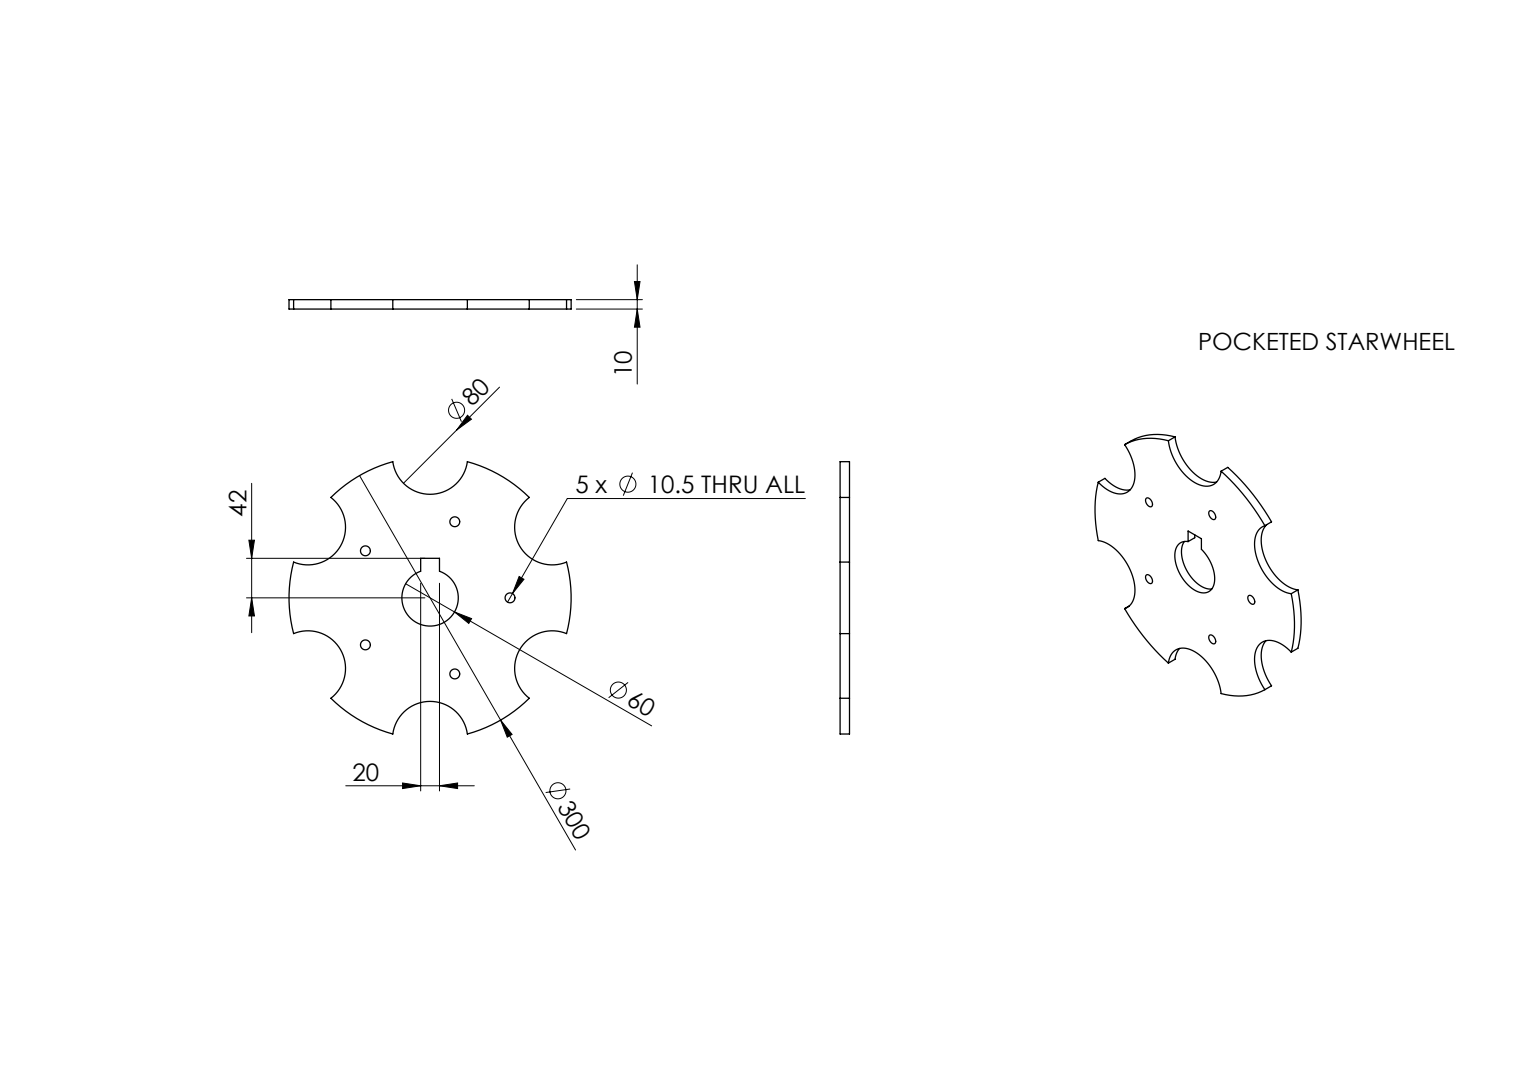
ISO-10303-21;
HEADER;
FILE_DESCRIPTION (('STEP AP214'),
    '1' );
FILE_NAME ('Pocketed Starwheel.step',
    '2026-10-23T05:12:30',
    ( '' ),
    ( '' ),
    'SwSTEP 2.0',
    'SolidWorks 2026',
    '' );
FILE_SCHEMA (( 'AUTOMOTIVE_DESIGN' ));
ENDSEC;

DATA;
#6=PRODUCT ( 'Pocketed Starwheel', 'Pocketed Starwheel', '', ( #881 ) ) ;
#8=EDGE_LOOP ( 'NONE', ( #780, #5698, #1230, #898 ) ) ;
#23=AXIS2_PLACEMENT_3D ( 'NONE', #6138, #4316, #7358 ) ;
#24=CARTESIAN_POINT ( 'NONE',  ( 129.9038105676649764, 75.00000000000153477, 10.00000000000000000 ) ) ;
#31=CIRCLE ( 'NONE', #2437, 40.00000000000001421 ) ;
#33=ORIENTED_EDGE ( 'NONE', *, *, #894, .F. ) ;
#38=PRODUCT_DEFINITION_FORMATION_WITH_SPECIFIED_SOURCE ( 'ANY', '', #6, .NOT_KNOWN. ) ;
#43=CARTESIAN_POINT ( 'NONE',  ( -68.76644452187024115, -49.96174644486060856, 10.00000000000000000 ) ) ;
#52=CARTESIAN_POINT ( 'NONE',  ( 0.000000000000000000, 0.000000000000000000, 0.000000000000000000 ) ) ;
#57=VERTEX_POINT ( 'NONE', #3381 ) ;
#59=DIRECTION ( 'NONE',  ( -1.000000000000000000, 0.000000000000000000, 0.000000000000000000 ) ) ;
#79=AXIS2_PLACEMENT_3D ( 'NONE', #1466, #7494, #2111 ) ;
#82=EDGE_CURVE ( 'NONE', #2245, #3533, #4731, .T. ) ;
#96=CARTESIAN_POINT ( 'NONE',  ( 85.00000000000000000, 9.720002580593245511E-13, 0.000000000000000000 ) ) ;
#104=DIRECTION ( 'NONE',  ( -0.000000000000000000, -0.000000000000000000, 1.000000000000000000 ) ) ;
#106=EDGE_LOOP ( 'NONE', ( #1599, #408, #5077, #4129 ) ) ;
#110=FACE_OUTER_BOUND ( 'NONE', #139, .T. ) ;
#114=CIRCLE ( 'NONE', #2185, 5.250000000000004441 ) ;
#135=CARTESIAN_POINT ( 'NONE',  ( 0.000000000000000000, 0.000000000000000000, 10.00000000000000000 ) ) ;
#138=EDGE_CURVE ( 'NONE', #7150, #5807, #1160, .T. ) ;
#139=EDGE_LOOP ( 'NONE', ( #4956, #6547, #3678, #7659 ) ) ;
#141=CARTESIAN_POINT ( 'NONE',  ( -39.64284999284935651, -144.6666666666667140, 10.00000000000000000 ) ) ;
#143=DIRECTION ( 'NONE',  ( -0.000000000000000000, -0.000000000000000000, 1.000000000000000000 ) ) ;
#146=CARTESIAN_POINT ( 'NONE',  ( 105.4635834177229299, 106.6650485055578770, 0.000000000000000000 ) ) ;
#161=SURFACE_STYLE_FILL_AREA ( #749 ) ;
#164=AXIS2_PLACEMENT_3D ( 'NONE', #7366, #2525, #6697 ) ;
#167=DIRECTION ( 'NONE',  ( 0.000000000000000000, 0.000000000000000000, 1.000000000000000000 ) ) ;
#175=DIRECTION ( 'NONE',  ( -1.000000000000000000, 0.000000000000000000, 0.000000000000000000 ) ) ;
#190=DIRECTION ( 'NONE',  ( 0.000000000000000000, -0.000000000000000000, -1.000000000000000000 ) ) ;
#195=ORIENTED_EDGE ( 'NONE', *, *, #3698, .F. ) ;
#202=DIRECTION ( 'NONE',  ( 1.000000000000000000, 0.000000000000000000, 0.000000000000000000 ) ) ;
#209=DIRECTION ( 'NONE',  ( 1.000000000000000000, 0.000000000000000000, 0.000000000000000000 ) ) ;
#215=EDGE_CURVE ( 'NONE', #5454, #5308, #3730, .T. ) ;
#220=ADVANCED_FACE ( 'NONE', ( #4830 ), #7323, .F. ) ;
#221=CIRCLE ( 'NONE', #3133, 5.250000000000004441 ) ;
#223=EDGE_CURVE ( 'NONE', #6783, #3903, #7702, .T. ) ;
#230=ORIENTED_EDGE ( 'NONE', *, *, #4072, .F. ) ;
#232=ORIENTED_EDGE ( 'NONE', *, *, #991, .T. ) ;
#239=LINE ( 'NONE', #274, #7501 ) ;
#240=DIRECTION ( 'NONE',  ( -0.000000000000000000, -0.000000000000000000, -1.000000000000000000 ) ) ;
#248=DIRECTION ( 'NONE',  ( -1.000000000000000000, 0.000000000000000000, 0.000000000000000000 ) ) ;
#255=ORIENTED_EDGE ( 'NONE', *, *, #5004, .T. ) ;
#260=DIRECTION ( 'NONE',  ( 0.000000000000000000, 0.000000000000000000, -1.000000000000000000 ) ) ;
#271=DIRECTION ( 'NONE',  ( 0.000000000000000000, 0.000000000000000000, 1.000000000000000000 ) ) ;
#274=CARTESIAN_POINT ( 'NONE',  ( 10.00000000000000000, 42.00000000000000000, 0.000000000000000000 ) ) ;
#277=AXIS2_PLACEMENT_3D ( 'NONE', #4146, #677, #1148 ) ;
#286=DIRECTION ( 'NONE',  ( -0.000000000000000000, -0.000000000000000000, 1.000000000000000000 ) ) ;
#289=DIRECTION ( 'NONE',  ( 0.000000000000000000, 0.000000000000000000, 1.000000000000000000 ) ) ;
#294=VERTEX_POINT ( 'NONE', #141 ) ;
#307=ORIENTED_EDGE ( 'NONE', *, *, #7076, .T. ) ;
#314=EDGE_CURVE ( 'NONE', #5791, #5558, #448, .T. ) ;
#325=FACE_BOUND ( 'NONE', #6779, .T. ) ;
#331=CARTESIAN_POINT ( 'NONE',  ( 0.000000000000000000, 0.000000000000000000, 0.000000000000000000 ) ) ;
#345=AXIS2_PLACEMENT_3D ( 'NONE', #357, #4696, #2348 ) ;
#348=FACE_OUTER_BOUND ( 'NONE', #4201, .T. ) ;
#354=EDGE_CURVE ( 'NONE', #6826, #2635, #830, .T. ) ;
#357=CARTESIAN_POINT ( 'NONE',  ( 129.9038105676665396, -74.99999999999882050, 10.00000000000000000 ) ) ;
#358=ADVANCED_FACE ( 'NONE', ( #4393 ), #7469, .F. ) ;
#361=AXIS2_PLACEMENT_3D ( 'NONE', #4667, #4589, #6527 ) ;
#364=CARTESIAN_POINT ( 'NONE',  ( -10.00000000000000000, 28.28427124746190202, 0.000000000000000000 ) ) ;
#373=VECTOR ( 'NONE', #6743, 1000.000000000000000 ) ;
#395=DIRECTION ( 'NONE',  ( 0.000000000000000000, 0.000000000000000000, -1.000000000000000000 ) ) ;
#402=CARTESIAN_POINT ( 'NONE',  ( -68.76644452187024115, -49.96174644486060856, 0.000000000000000000 ) ) ;
#407=CIRCLE ( 'NONE', #7096, 5.250000000000004441 ) ;
#408=ORIENTED_EDGE ( 'NONE', *, *, #3368, .T. ) ;
#424=ORIENTED_EDGE ( 'NONE', *, *, #5929, .F. ) ;
#430=DIRECTION ( 'NONE',  ( 1.000000000000000000, 0.000000000000000000, 0.000000000000000000 ) ) ;
#437=CARTESIAN_POINT ( 'NONE',  ( 0.000000000000000000, 0.000000000000000000, 10.00000000000000000 ) ) ;
#448=CIRCLE ( 'NONE', #4230, 40.00000000000000711 ) ;
#449=ORIENTED_EDGE ( 'NONE', *, *, #7450, .F. ) ;
#450=ORIENTED_EDGE ( 'NONE', *, *, #4469, .T. ) ;
#460=ADVANCED_FACE ( 'NONE', ( #2627 ), #6369, .F. ) ;
#466=CARTESIAN_POINT ( 'NONE',  ( 26.26644452187053957, 80.83980388508807380, 10.00000000000000000 ) ) ;
#472=DIRECTION ( 'NONE',  ( 0.000000000000000000, 0.000000000000000000, 1.000000000000000000 ) ) ;
#495=CARTESIAN_POINT ( 'NONE',  ( 0.000000000000000000, 0.000000000000000000, 0.000000000000000000 ) ) ;
#497=CARTESIAN_POINT ( 'NONE',  ( 31.51644452187053602, 80.83980388508807380, 10.00000000000000000 ) ) ;
#508=EDGE_CURVE ( 'NONE', #57, #5308, #1029, .T. ) ;
#510=ORIENTED_EDGE ( 'NONE', *, *, #6970, .F. ) ;
#519=ORIENTED_EDGE ( 'NONE', *, *, #5812, .T. ) ;
#522=CARTESIAN_POINT ( 'NONE',  ( 39.64284999284934941, 144.6666666666667140, 5.000000000000000000 ) ) ;
#529=EDGE_CURVE ( 'NONE', #6340, #6348, #6500, .T. ) ;
#554=CYLINDRICAL_SURFACE ( 'NONE', #7508, 150.0000000000000568 ) ;
#555=DIRECTION ( 'NONE',  ( -0.000000000000000000, -0.000000000000000000, 1.000000000000000000 ) ) ;
#556=MECHANICAL_DESIGN_GEOMETRIC_PRESENTATION_REPRESENTATION('',(#1054),#799);
#570=DIRECTION ( 'NONE',  ( 0.000000000000000000, 0.000000000000000000, 1.000000000000000000 ) ) ;
#580=CARTESIAN_POINT ( 'NONE',  ( 10.00000000000000000, 28.28427124746190202, 0.000000000000000000 ) ) ;
#589=VERTEX_POINT ( 'NONE', #4784 ) ;
#590=DIRECTION ( 'NONE',  ( 0.000000000000000000, -0.000000000000000000, -1.000000000000000000 ) ) ;
#614=VECTOR ( 'NONE', #286, 1000.000000000000000 ) ;
#624=ORIENTED_EDGE ( 'NONE', *, *, #2405, .T. ) ;
#631=CARTESIAN_POINT ( 'NONE',  ( 0.000000000000000000, -150.0000000000000568, 10.00000000000000000 ) ) ;
#634=ORIENTED_EDGE ( 'NONE', *, *, #7223, .T. ) ;
#637=SHAPE_REPRESENTATION ( 'Pocketed Starwheel', ( #7485 ), #2086 ) ;
#642=EDGE_LOOP ( 'NONE', ( #3769, #1334 ) ) ;
#653=CARTESIAN_POINT ( 'NONE',  ( -39.64284999284935651, 144.6666666666667140, 10.00000000000000000 ) ) ;
#659=ORIENTED_EDGE ( 'NONE', *, *, #7204, .T. ) ;
#663=ORIENTED_EDGE ( 'NONE', *, *, #7369, .T. ) ;
#664=DIRECTION ( 'NONE',  ( 1.000000000000000000, 0.000000000000000000, 0.000000000000000000 ) ) ;
#665=AXIS2_PLACEMENT_3D ( 'NONE', #4618, #472, #430 ) ;
#677=DIRECTION ( 'NONE',  ( -0.000000000000000000, -0.000000000000000000, 1.000000000000000000 ) ) ;
#685=DIRECTION ( 'NONE',  ( 0.000000000000000000, 0.000000000000000000, 1.000000000000000000 ) ) ;
#698=ORIENTED_EDGE ( 'NONE', *, *, #2750, .F. ) ;
#699=VERTEX_POINT ( 'NONE', #1951 ) ;
#708=ORIENTED_EDGE ( 'NONE', *, *, #3264, .T. ) ;
#714=AXIS2_PLACEMENT_3D ( 'NONE', #3882, #3330, #2041 ) ;
#721=CARTESIAN_POINT ( 'NONE',  ( 89.90381056766497636, 75.00000000000153477, 0.000000000000000000 ) ) ;
#722=LINE ( 'NONE', #6945, #1174 ) ;
#740=LINE ( 'NONE', #1932, #373 ) ;
#742=LINE ( 'NONE', #6704, #5973 ) ;
#749=FILL_AREA_STYLE ('',( #5523 ) ) ;
#753=VECTOR ( 'NONE', #260, 1000.000000000000000 ) ;
#754=EDGE_CURVE ( 'NONE', #7338, #2067, #1723, .T. ) ;
#755=EDGE_LOOP ( 'NONE', ( #5490, #6461, #7212, #2166 ) ) ;
#759=DIRECTION ( 'NONE',  ( 0.000000000000000000, 0.000000000000000000, -1.000000000000000000 ) ) ;
#760=CIRCLE ( 'NONE', #7682, 40.00000000000001421 ) ;
#780=ORIENTED_EDGE ( 'NONE', *, *, #6297, .F. ) ;
#784=CARTESIAN_POINT ( 'NONE',  ( -74.01644452187068168, 49.96174644486002592, 0.000000000000000000 ) ) ;
#795=EDGE_CURVE ( 'NONE', #3391, #5308, #239, .T. ) ;
#797=ORIENTED_EDGE ( 'NONE', *, *, #4469, .F. ) ;
#799=( GEOMETRIC_REPRESENTATION_CONTEXT ( 3 ) GLOBAL_UNCERTAINTY_ASSIGNED_CONTEXT ( ( #6208 ) ) GLOBAL_UNIT_ASSIGNED_CONTEXT ( ( #6695, #3035, #7249 ) ) REPRESENTATION_CONTEXT ( 'NONE', 'WORKASPACE' ) );
#821=CARTESIAN_POINT ( 'NONE',  ( 0.000000000000000000, 0.000000000000000000, 10.00000000000000000 ) ) ;
#827=DIRECTION ( 'NONE',  ( -0.4999999999999918954, -0.8660254037844432595, 0.000000000000000000 ) ) ;
#830=CIRCLE ( 'NONE', #3608, 150.0000000000000568 ) ;
#832=ORIENTED_EDGE ( 'NONE', *, *, #529, .T. ) ;
#848=EDGE_LOOP ( 'NONE', ( #5860, #2174 ) ) ;
#853=ORIENTED_EDGE ( 'NONE', *, *, #3653, .F. ) ;
#870=DIRECTION ( 'NONE',  ( -1.000000000000000000, 0.000000000000000000, 0.000000000000000000 ) ) ;
#871=CARTESIAN_POINT ( 'NONE',  ( -145.1064334105735725, 38.00161816110974655, 0.000000000000000000 ) ) ;
#881=PRODUCT_CONTEXT ( 'NONE', #6213, 'mechanical' ) ;
#889=AXIS2_PLACEMENT_3D ( 'NONE', #4293, #7335, #1330 ) ;
#894=EDGE_CURVE ( 'NONE', #5165, #4732, #5114, .T. ) ;
#898=ORIENTED_EDGE ( 'NONE', *, *, #1531, .T. ) ;
#924=VERTEX_POINT ( 'NONE', #7571 ) ;
#938=EDGE_CURVE ( 'NONE', #2235, #5183, #3616, .T. ) ;
#944=DIRECTION ( 'NONE',  ( 1.000000000000000000, 0.000000000000000000, 0.000000000000000000 ) ) ;
#949=AXIS2_PLACEMENT_3D ( 'NONE', #2122, #1512, #209 ) ;
#954=LINE ( 'NONE', #522, #5751 ) ;
#955=DIRECTION ( 'NONE',  ( -0.000000000000000000, 0.000000000000000000, -1.000000000000000000 ) ) ;
#959=AXIS2_PLACEMENT_3D ( 'NONE', #4354, #6771, #1592 ) ;
#963=ORIENTED_EDGE ( 'NONE', *, *, #7549, .T. ) ;
#964=AXIS2_PLACEMENT_3D ( 'NONE', #6067, #143, #1920 ) ;
#969=DIRECTION ( 'NONE',  ( -1.000000000000000000, 0.000000000000000000, 0.000000000000000000 ) ) ;
#976=CARTESIAN_POINT ( 'NONE',  ( 26.26644452187122170, -80.83980388508783221, 0.000000000000000000 ) ) ;
#985=DIRECTION ( 'NONE',  ( 0.000000000000000000, 0.000000000000000000, 1.000000000000000000 ) ) ;
#989=VERTEX_POINT ( 'NONE', #7694 ) ;
#991=EDGE_CURVE ( 'NONE', #5791, #3509, #1093, .T. ) ;
#993=AXIS2_PLACEMENT_3D ( 'NONE', #7133, #4168, #3502 ) ;
#1006=CARTESIAN_POINT ( 'NONE',  ( -10.00000000000000000, 0.000000000000000000, 10.00000000000000000 ) ) ;
#1017=CARTESIAN_POINT ( 'NONE',  ( -129.9038105676659995, 74.99999999999971578, 10.00000000000000000 ) ) ;
#1019=ORIENTED_EDGE ( 'NONE', *, *, #5521, .F. ) ;
#1023=DIRECTION ( 'NONE',  ( 1.000000000000000000, 0.000000000000000000, 0.000000000000000000 ) ) ;
#1024=AXIS2_PLACEMENT_3D ( 'NONE', #7353, #6917, #1352 ) ;
#1029=LINE ( 'NONE', #5298, #7628 ) ;
#1032=EDGE_CURVE ( 'NONE', #7478, #6571, #4999, .T. ) ;
#1038=ADVANCED_FACE ( 'NONE', ( #4142 ), #554, .T. ) ;
#1041=ORIENTED_EDGE ( 'NONE', *, *, #1937, .F. ) ;
#1054=STYLED_ITEM('',(#7823),#5726);
#1060=CYLINDRICAL_SURFACE ( 'NONE', #6349, 40.00000000000000711 ) ;
#1065=CARTESIAN_POINT ( 'NONE',  ( -129.9038105676659995, 74.99999999999971578, 0.000000000000000000 ) ) ;
#1070=ORIENTED_EDGE ( 'NONE', *, *, #3698, .T. ) ;
#1092=ORIENTED_EDGE ( 'NONE', *, *, #3497, .T. ) ;
#1093=CIRCLE ( 'NONE', #5251, 150.0000000000000568 ) ;
#1096=DIRECTION ( 'NONE',  ( -1.000000000000000000, 0.000000000000000000, 0.000000000000000000 ) ) ;
#1109=EDGE_LOOP ( 'NONE', ( #3754, #7137 ) ) ;
#1110=ORIENTED_EDGE ( 'NONE', *, *, #2750, .T. ) ;
#1115=FACE_BOUND ( 'NONE', #1109, .T. ) ;
#1125=CARTESIAN_POINT ( 'NONE',  ( -63.51644452187023404, -49.96174644486060856, 0.000000000000000000 ) ) ;
#1129=VECTOR ( 'NONE', #4406, 1000.000000000000000 ) ;
#1137=ADVANCED_FACE ( 'NONE', ( #2625, #7467, #3917, #2079, #325, #7391, #4472 ), #5581, .T. ) ;
#1143=VECTOR ( 'NONE', #1204, 1000.000000000000000 ) ;
#1145=DIRECTION ( 'NONE',  ( -0.000000000000000000, -0.000000000000000000, 1.000000000000000000 ) ) ;
#1148=DIRECTION ( 'NONE',  ( 1.000000000000000000, 0.000000000000000000, 0.000000000000000000 ) ) ;
#1149=ORIENTED_EDGE ( 'NONE', *, *, #1937, .T. ) ;
#1154=( NAMED_UNIT ( * ) SI_UNIT ( $, .STERADIAN. ) SOLID_ANGLE_UNIT ( ) );
#1157=CIRCLE ( 'NONE', #1802, 5.250000000000004441 ) ;
#1160=CIRCLE ( 'NONE', #7322, 150.0000000000000568 ) ;
#1163=DIRECTION ( 'NONE',  ( 0.000000000000000000, 0.000000000000000000, 1.000000000000000000 ) ) ;
#1174=VECTOR ( 'NONE', #3724, 1000.000000000000000 ) ;
#1192=ADVANCED_FACE ( 'NONE', ( #6920 ), #5730, .F. ) ;
#1194=VERTEX_POINT ( 'NONE', #6482 ) ;
#1204=DIRECTION ( 'NONE',  ( 1.000000000000000000, 0.000000000000000000, -0.000000000000000000 ) ) ;
#1210=CYLINDRICAL_SURFACE ( 'NONE', #993, 150.0000000000000568 ) ;
#1215=DIRECTION ( 'NONE',  ( 0.000000000000000000, -1.000000000000000000, 0.000000000000000000 ) ) ;
#1219=VERTEX_POINT ( 'NONE', #7035 ) ;
#1230=ORIENTED_EDGE ( 'NONE', *, *, #6643, .T. ) ;
#1233=AXIS2_PLACEMENT_3D ( 'NONE', #6332, #3600, #6598 ) ;
#1234=DIRECTION ( 'NONE',  ( 1.000000000000000000, 0.000000000000000000, 0.000000000000000000 ) ) ;
#1241=CARTESIAN_POINT ( 'NONE',  ( 0.000000000000000000, 0.000000000000000000, 10.00000000000000000 ) ) ;
#1244=CARTESIAN_POINT ( 'NONE',  ( -68.76644452187024115, -49.96174644486060856, 0.000000000000000000 ) ) ;
#1249=CARTESIAN_POINT ( 'NONE',  ( 26.26644452187122170, -80.83980388508783221, 10.00000000000000000 ) ) ;
#1254=EDGE_LOOP ( 'NONE', ( #4422, #6940 ) ) ;
#1260=ORIENTED_EDGE ( 'NONE', *, *, #5004, .F. ) ;
#1275=EDGE_LOOP ( 'NONE', ( #7512, #1260, #4727, #6662 ) ) ;
#1278=EDGE_CURVE ( 'NONE', #2635, #6563, #954, .T. ) ;
#1292=CARTESIAN_POINT ( 'NONE',  ( -10.00000000000000000, 42.00000000000000000, 0.000000000000000000 ) ) ;
#1297=ORIENTED_EDGE ( 'NONE', *, *, #1032, .F. ) ;
#1301=CARTESIAN_POINT ( 'NONE',  ( 0.000000000000000000, 0.000000000000000000, 0.000000000000000000 ) ) ;
#1304=LINE ( 'NONE', #4815, #2060 ) ;
#1312=CARTESIAN_POINT ( 'NONE',  ( 26.26644452187122170, -80.83980388508783221, 10.00000000000000000 ) ) ;
#1313=UNCERTAINTY_MEASURE_WITH_UNIT (LENGTH_MEASURE( 1.000000000000000082E-05 ), #3527, 'distance_accuracy_value', 'NONE');
#1328=ORIENTED_EDGE ( 'NONE', *, *, #2081, .F. ) ;
#1330=DIRECTION ( 'NONE',  ( -1.000000000000000000, 0.000000000000000000, 0.000000000000000000 ) ) ;
#1334=ORIENTED_EDGE ( 'NONE', *, *, #7076, .F. ) ;
#1339=EDGE_CURVE ( 'NONE', #6807, #5511, #5809, .T. ) ;
#1343=ORIENTED_EDGE ( 'NONE', *, *, #508, .F. ) ;
#1349=DIRECTION ( 'NONE',  ( 1.000000000000000000, 0.000000000000000000, 0.000000000000000000 ) ) ;
#1352=DIRECTION ( 'NONE',  ( 1.000000000000000000, 0.000000000000000000, 0.000000000000000000 ) ) ;
#1366=DIRECTION ( 'NONE',  ( -0.000000000000000000, 0.000000000000000000, -1.000000000000000000 ) ) ;
#1375=EDGE_CURVE ( 'NONE', #5121, #6571, #7635, .T. ) ;
#1385=ADVANCED_FACE ( 'NONE', ( #2250 ), #7086, .F. ) ;
#1390=VECTOR ( 'NONE', #555, 1000.000000000000000 ) ;
#1403=ORIENTED_EDGE ( 'NONE', *, *, #2848, .T. ) ;
#1407=DIRECTION ( 'NONE',  ( 0.000000000000000000, 0.000000000000000000, 1.000000000000000000 ) ) ;
#1417=AXIS2_PLACEMENT_3D ( 'NONE', #4268, #1952, #759 ) ;
#1421=DIRECTION ( 'NONE',  ( -0.000000000000000000, -0.000000000000000000, 1.000000000000000000 ) ) ;
#1422=DIRECTION ( 'NONE',  ( -0.000000000000000000, 0.000000000000000000, 1.000000000000000000 ) ) ;
#1426=DIRECTION ( 'NONE',  ( 0.000000000000000000, 0.000000000000000000, 1.000000000000000000 ) ) ;
#1429=VECTOR ( 'NONE', #190, 1000.000000000000000 ) ;
#1430=AXIS2_PLACEMENT_3D ( 'NONE', #4502, #985, #870 ) ;
#1434=FACE_OUTER_BOUND ( 'NONE', #4506, .T. ) ;
#1440=ORIENTED_EDGE ( 'NONE', *, *, #7369, .F. ) ;
#1450=CYLINDRICAL_SURFACE ( 'NONE', #3082, 40.00000000000000711 ) ;
#1454=ORIENTED_EDGE ( 'NONE', *, *, #2012, .T. ) ;
#1466=CARTESIAN_POINT ( 'NONE',  ( 129.9038105676649764, 75.00000000000153477, 0.000000000000000000 ) ) ;
#1467=DIRECTION ( 'NONE',  ( 1.000000000000000000, 0.000000000000000000, 0.000000000000000000 ) ) ;
#1469=DIRECTION ( 'NONE',  ( 1.000000000000000000, 0.000000000000000000, 0.000000000000000000 ) ) ;
#1476=CYLINDRICAL_SURFACE ( 'NONE', #2701, 150.0000000000000568 ) ;
#1484=CIRCLE ( 'NONE', #5392, 150.0000000000000568 ) ;
#1501=DIRECTION ( 'NONE',  ( -0.000000000000000000, -0.000000000000000000, 1.000000000000000000 ) ) ;
#1503=AXIS2_PLACEMENT_3D ( 'NONE', #3151, #4398, #5627 ) ;
#1508=CARTESIAN_POINT ( 'NONE',  ( 145.1064334105730893, 38.00161816111175739, 10.00000000000000000 ) ) ;
#1512=DIRECTION ( 'NONE',  ( -0.000000000000000000, -0.000000000000000000, 1.000000000000000000 ) ) ;
#1514=CARTESIAN_POINT ( 'NONE',  ( -10.00000000000000000, 42.00000000000000000, 0.000000000000000000 ) ) ;
#1524=ORIENTED_EDGE ( 'NONE', *, *, #2927, .F. ) ;
#1526=VERTEX_POINT ( 'NONE', #7284 ) ;
#1530=FACE_OUTER_BOUND ( 'NONE', #2638, .T. ) ;
#1531=EDGE_CURVE ( 'NONE', #1219, #5930, #7143, .T. ) ;
#1533=EDGE_LOOP ( 'NONE', ( #6280, #3924 ) ) ;
#1541=AXIS2_PLACEMENT_3D ( 'NONE', #3396, #7060, #944 ) ;
#1544=DIRECTION ( 'NONE',  ( -0.000000000000000000, -0.000000000000000000, 1.000000000000000000 ) ) ;
#1558=ORIENTED_EDGE ( 'NONE', *, *, #3708, .T. ) ;
#1572=VERTEX_POINT ( 'NONE', #653 ) ;
#1585=LINE ( 'NONE', #3876, #6474 ) ;
#1592=DIRECTION ( 'NONE',  ( 1.000000000000000000, 0.000000000000000000, 0.000000000000000000 ) ) ;
#1598=LINE ( 'NONE', #3376, #1959 ) ;
#1599=ORIENTED_EDGE ( 'NONE', *, *, #1339, .T. ) ;
#1600=ORIENTED_EDGE ( 'NONE', *, *, #6442, .F. ) ;
#1617=ADVANCED_FACE ( 'NONE', ( #4396 ), #3187, .F. ) ;
#1626=DIRECTION ( 'NONE',  ( 1.000000000000000000, 0.000000000000000000, 0.000000000000000000 ) ) ;
#1628=VECTOR ( 'NONE', #4680, 1000.000000000000000 ) ;
#1639=ORIENTED_EDGE ( 'NONE', *, *, #6385, .F. ) ;
#1648=CYLINDRICAL_SURFACE ( 'NONE', #4078, 150.0000000000000568 ) ;
#1651=VERTEX_POINT ( 'NONE', #5029 ) ;
#1656=CARTESIAN_POINT ( 'NONE',  ( 26.26644452187053957, 80.83980388508807380, 0.000000000000000000 ) ) ;
#1662=DIRECTION ( 'NONE',  ( 0.4999999999999979461, 0.8660254037844398178, 0.000000000000000000 ) ) ;
#1663=CARTESIAN_POINT ( 'NONE',  ( 129.9038105676649764, 75.00000000000153477, 10.00000000000000000 ) ) ;
#1673=( LENGTH_UNIT ( ) NAMED_UNIT ( * ) SI_UNIT ( .MILLI., .METRE. ) );
#1682=EDGE_LOOP ( 'NONE', ( #5830, #1092, #2508, #3562 ) ) ;
#1690=FACE_OUTER_BOUND ( 'NONE', #6336, .T. ) ;
#1695=AXIS2_PLACEMENT_3D ( 'NONE', #5613, #2620, #202 ) ;
#1697=DIRECTION ( 'NONE',  ( -0.000000000000000000, -0.000000000000000000, -1.000000000000000000 ) ) ;
#1704=DIRECTION ( 'NONE',  ( 1.000000000000000000, 0.000000000000000000, 0.000000000000000000 ) ) ;
#1717=DIRECTION ( 'NONE',  ( 1.000000000000000000, 0.000000000000000000, 0.000000000000000000 ) ) ;
#1723=CIRCLE ( 'NONE', #79, 40.00000000000000000 ) ;
#1726=ORIENTED_EDGE ( 'NONE', *, *, #2687, .T. ) ;
#1735=FACE_OUTER_BOUND ( 'NONE', #2463, .T. ) ;
#1736=CARTESIAN_POINT ( 'NONE',  ( 0.000000000000000000, 0.000000000000000000, 10.00000000000000000 ) ) ;
#1744=ORIENTED_EDGE ( 'NONE', *, *, #5346, .T. ) ;
#1752=DIRECTION ( 'NONE',  ( -0.000000000000000000, -0.000000000000000000, -1.000000000000000000 ) ) ;
#1760=ORIENTED_EDGE ( 'NONE', *, *, #1820, .T. ) ;
#1761=DIRECTION ( 'NONE',  ( 0.000000000000000000, 1.000000000000000000, 0.000000000000000000 ) ) ;
#1769=ORIENTED_EDGE ( 'NONE', *, *, #5929, .T. ) ;
#1790=AXIS2_PLACEMENT_3D ( 'NONE', #3511, #4728, #4769 ) ;
#1793=FACE_OUTER_BOUND ( 'NONE', #7600, .T. ) ;
#1802=AXIS2_PLACEMENT_3D ( 'NONE', #96, #2515, #4908 ) ;
#1804=ORIENTED_EDGE ( 'NONE', *, *, #5568, .T. ) ;
#1807=DIRECTION ( 'NONE',  ( -0.000000000000000000, -0.000000000000000000, 1.000000000000000000 ) ) ;
#1812=LINE ( 'NONE', #6030, #4780 ) ;
#1820=EDGE_CURVE ( 'NONE', #4328, #2865, #221, .T. ) ;
#1822=AXIS2_PLACEMENT_3D ( 'NONE', #631, #1407, #7483 ) ;
#1825=ORIENTED_EDGE ( 'NONE', *, *, #5000, .F. ) ;
#1828=AXIS2_PLACEMENT_3D ( 'NONE', #331, #289, #5030 ) ;
#1829=( GEOMETRIC_REPRESENTATION_CONTEXT ( 3 ) GLOBAL_UNCERTAINTY_ASSIGNED_CONTEXT ( ( #5575 ) ) GLOBAL_UNIT_ASSIGNED_CONTEXT ( ( #1673, #4456, #2724 ) ) REPRESENTATION_CONTEXT ( 'NONE', 'WORKASPACE' ) );
#1861=EDGE_LOOP ( 'NONE', ( #4404, #1558 ) ) ;
#1866=CYLINDRICAL_SURFACE ( 'NONE', #277, 5.250000000000004441 ) ;
#1870=CIRCLE ( 'NONE', #3126, 40.00000000000000711 ) ;
#1884=AXIS2_PLACEMENT_3D ( 'NONE', #5222, #5300, #2860 ) ;
#1886=DIRECTION ( 'NONE',  ( 1.000000000000000000, 0.000000000000000000, 0.000000000000000000 ) ) ;
#1911=DIRECTION ( 'NONE',  ( 0.000000000000000000, 0.000000000000000000, 1.000000000000000000 ) ) ;
#1917=DIRECTION ( 'NONE',  ( 0.000000000000000000, 0.000000000000000000, -1.000000000000000000 ) ) ;
#1920=DIRECTION ( 'NONE',  ( 1.000000000000000000, 0.000000000000000000, 0.000000000000000000 ) ) ;
#1925=EDGE_LOOP ( 'NONE', ( #634, #519, #6187, #1744, #3454, #6306 ) ) ;
#1926=AXIS2_PLACEMENT_3D ( 'NONE', #4028, #6440, #1023 ) ;
#1932=CARTESIAN_POINT ( 'NONE',  ( -105.4635834177243936, 106.6650485055563990, 5.000000000000000000 ) ) ;
#1937=EDGE_CURVE ( 'NONE', #6826, #2604, #7650, .T. ) ;
#1940=ORIENTED_EDGE ( 'NONE', *, *, #2645, .F. ) ;
#1942=DIRECTION ( 'NONE',  ( 1.000000000000000000, 0.000000000000000000, 0.000000000000000000 ) ) ;
#1951=CARTESIAN_POINT ( 'NONE',  ( 39.64284999284935651, -144.6666666666667140, 10.00000000000000000 ) ) ;
#1952=DIRECTION ( 'NONE',  ( 1.000000000000000000, 0.000000000000000000, 0.000000000000000000 ) ) ;
#1959=VECTOR ( 'NONE', #4709, 1000.000000000000000 ) ;
#1962=CARTESIAN_POINT ( 'NONE',  ( -129.9038105676659995, 74.99999999999971578, 10.00000000000000000 ) ) ;
#1986=DIRECTION ( 'NONE',  ( 0.000000000000000000, 0.000000000000000000, 1.000000000000000000 ) ) ;
#1989=LINE ( 'NONE', #6240, #2389 ) ;
#1991=ORIENTED_EDGE ( 'NONE', *, *, #2405, .F. ) ;
#1997=LINE ( 'NONE', #2586, #3811 ) ;
#2010=ORIENTED_EDGE ( 'NONE', *, *, #2687, .F. ) ;
#2012=EDGE_CURVE ( 'NONE', #6651, #4919, #7524, .T. ) ;
#2019=AXIS2_PLACEMENT_3D ( 'NONE', #1736, #4836, #4209 ) ;
#2037=EDGE_CURVE ( 'NONE', #1572, #2635, #1870, .T. ) ;
#2038=EDGE_LOOP ( 'NONE', ( #1343, #7627, #6479, #3190, #708, #7738 ) ) ;
#2041=DIRECTION ( 'NONE',  ( 1.000000000000000000, 0.000000000000000000, -0.000000000000000000 ) ) ;
#2053=CARTESIAN_POINT ( 'NONE',  ( 26.26644452187122170, -80.83980388508783221, 10.00000000000000000 ) ) ;
#2055=CARTESIAN_POINT ( 'NONE',  ( 129.9038105676665396, -74.99999999999882050, 10.00000000000000000 ) ) ;
#2056=AXIS2_PLACEMENT_3D ( 'NONE', #7616, #5215, #1626 ) ;
#2059=ORIENTED_EDGE ( 'NONE', *, *, #6746, .T. ) ;
#2060=VECTOR ( 'NONE', #7733, 1000.000000000000000 ) ;
#2066=AXIS2_PLACEMENT_3D ( 'NONE', #4110, #6014, #5422 ) ;
#2067=VERTEX_POINT ( 'NONE', #6133 ) ;
#2079=FACE_BOUND ( 'NONE', #642, .T. ) ;
#2081=EDGE_CURVE ( 'NONE', #699, #1651, #1484, .T. ) ;
#2086=( GEOMETRIC_REPRESENTATION_CONTEXT ( 3 ) GLOBAL_UNCERTAINTY_ASSIGNED_CONTEXT ( ( #1313 ) ) GLOBAL_UNIT_ASSIGNED_CONTEXT ( ( #3527, #4891, #1154 ) ) REPRESENTATION_CONTEXT ( 'NONE', 'WORKASPACE' ) );
#2106=AXIS2_PLACEMENT_3D ( 'NONE', #4658, #3518, #7027 ) ;
#2107=CARTESIAN_POINT ( 'NONE',  ( 105.4635834177229157, 106.6650485055578770, 10.00000000000000000 ) ) ;
#2111=DIRECTION ( 'NONE',  ( 0.5000000000000101030, -0.8660254037844328234, 0.000000000000000000 ) ) ;
#2117=DIRECTION ( 'NONE',  ( -0.4999999999999918954, -0.8660254037844432595, 0.000000000000000000 ) ) ;
#2122=CARTESIAN_POINT ( 'NONE',  ( 0.000000000000000000, 0.000000000000000000, 0.000000000000000000 ) ) ;
#2131=AXIS2_PLACEMENT_3D ( 'NONE', #1312, #3100, #2479 ) ;
#2145=DIRECTION ( 'NONE',  ( 0.000000000000000000, 0.000000000000000000, 1.000000000000000000 ) ) ;
#2150=CARTESIAN_POINT ( 'NONE',  ( 21.01644452187054313, 80.83980388508807380, 10.00000000000000000 ) ) ;
#2152=AXIS2_PLACEMENT_3D ( 'NONE', #1656, #7098, #5280 ) ;
#2160=DIRECTION ( 'NONE',  ( 1.000000000000000000, 0.000000000000000000, 0.000000000000000000 ) ) ;
#2166=ORIENTED_EDGE ( 'NONE', *, *, #4271, .F. ) ;
#2172=LINE ( 'NONE', #2211, #753 ) ;
#2174=ORIENTED_EDGE ( 'NONE', *, *, #4072, .T. ) ;
#2180=VECTOR ( 'NONE', #7427, 1000.000000000000000 ) ;
#2185=AXIS2_PLACEMENT_3D ( 'NONE', #2196, #7546, #2160 ) ;
#2196=CARTESIAN_POINT ( 'NONE',  ( 85.00000000000000000, 9.720002580593245511E-13, 10.00000000000000000 ) ) ;
#2211=CARTESIAN_POINT ( 'NONE',  ( -39.64284999284934941, -144.6666666666667140, 5.000000000000000000 ) ) ;
#2229=ORIENTED_EDGE ( 'NONE', *, *, #3702, .T. ) ;
#2231=CARTESIAN_POINT ( 'NONE',  ( 79.75000000000000000, 9.726431976288768917E-13, 10.00000000000000000 ) ) ;
#2235=VERTEX_POINT ( 'NONE', #871 ) ;
#2245=VERTEX_POINT ( 'NONE', #6363 ) ;
#2250=FACE_OUTER_BOUND ( 'NONE', #4663, .T. ) ;
#2252=CARTESIAN_POINT ( 'NONE',  ( 0.000000000000000000, 0.000000000000000000, 10.00000000000000000 ) ) ;
#2256=ORIENTED_EDGE ( 'NONE', *, *, #6553, .T. ) ;
#2269=DIRECTION ( 'NONE',  ( 1.000000000000000000, 0.000000000000000000, 0.000000000000000000 ) ) ;
#2282=ORIENTED_EDGE ( 'NONE', *, *, #5521, .T. ) ;
#2285=ORIENTED_EDGE ( 'NONE', *, *, #6258, .F. ) ;
#2290=CIRCLE ( 'NONE', #1790, 40.00000000000000000 ) ;
#2299=CARTESIAN_POINT ( 'NONE',  ( -68.76644452187068168, 49.96174644486002592, 10.00000000000000000 ) ) ;
#2301=CARTESIAN_POINT ( 'NONE',  ( -105.4635834177243794, 106.6650485055563990, 0.000000000000000000 ) ) ;
#2313=ORIENTED_EDGE ( 'NONE', *, *, #5477, .F. ) ;
#2322=CYLINDRICAL_SURFACE ( 'NONE', #361, 30.00000000000000000 ) ;
#2325=LINE ( 'NONE', #5778, #4840 ) ;
#2346=DIRECTION ( 'NONE',  ( 1.000000000000000000, 0.000000000000000000, 0.000000000000000000 ) ) ;
#2348=DIRECTION ( 'NONE',  ( -0.4999999999999918954, -0.8660254037844432595, 0.000000000000000000 ) ) ;
#2356=CARTESIAN_POINT ( 'NONE',  ( 0.000000000000000000, 0.000000000000000000, 0.000000000000000000 ) ) ;
#2374=DIRECTION ( 'NONE',  ( -0.000000000000000000, -0.000000000000000000, -1.000000000000000000 ) ) ;
#2377=EDGE_LOOP ( 'NONE', ( #6050, #3200, #4210, #6603 ) ) ;
#2386=CARTESIAN_POINT ( 'NONE',  ( 10.00000000000000000, 42.00000000000000000, 0.000000000000000000 ) ) ;
#2389=VECTOR ( 'NONE', #6198, 1000.000000000000000 ) ;
#2405=EDGE_CURVE ( 'NONE', #3290, #1651, #4132, .T. ) ;
#2415=EDGE_CURVE ( 'NONE', #2235, #5791, #3401, .T. ) ;
#2416=ORIENTED_EDGE ( 'NONE', *, *, #754, .T. ) ;
#2437=AXIS2_PLACEMENT_3D ( 'NONE', #3325, #5727, #2117 ) ;
#2439=ORIENTED_EDGE ( 'NONE', *, *, #3702, .F. ) ;
#2452=ORIENTED_EDGE ( 'NONE', *, *, #6406, .F. ) ;
#2455=AXIS2_PLACEMENT_3D ( 'NONE', #4054, #5878, #4178 ) ;
#2458=ADVANCED_FACE ( 'NONE', ( #1793 ), #4814, .F. ) ;
#2463=EDGE_LOOP ( 'NONE', ( #3605, #4352, #6627, #3263 ) ) ;
#2467=DIRECTION ( 'NONE',  ( -0.000000000000000000, -0.000000000000000000, 1.000000000000000000 ) ) ;
#2479=DIRECTION ( 'NONE',  ( 1.000000000000000000, 0.000000000000000000, 0.000000000000000000 ) ) ;
#2486=DIRECTION ( 'NONE',  ( 0.000000000000000000, 0.000000000000000000, -1.000000000000000000 ) ) ;
#2489=CARTESIAN_POINT ( 'NONE',  ( -129.9038105676655164, -75.00000000000063949, 0.000000000000000000 ) ) ;
#2491=VERTEX_POINT ( 'NONE', #5487 ) ;
#2508=ORIENTED_EDGE ( 'NONE', *, *, #6346, .T. ) ;
#2515=DIRECTION ( 'NONE',  ( -0.000000000000000000, -0.000000000000000000, 1.000000000000000000 ) ) ;
#2525=DIRECTION ( 'NONE',  ( 0.000000000000000000, 0.000000000000000000, 1.000000000000000000 ) ) ;
#2526=ORIENTED_EDGE ( 'NONE', *, *, #3708, .F. ) ;
#2530=PLANE ( 'NONE',  #4798 ) ;
#2567=VECTOR ( 'NONE', #1501, 1000.000000000000000 ) ;
#2569=EDGE_LOOP ( 'NONE', ( #6928, #1769, #1804, #3902 ) ) ;
#2577=CIRCLE ( 'NONE', #164, 150.0000000000000568 ) ;
#2580=AXIS2_PLACEMENT_3D ( 'NONE', #52, #167, #5456 ) ;
#2586=CARTESIAN_POINT ( 'NONE',  ( -74.01644452187024115, -49.96174644486060856, 10.00000000000000000 ) ) ;
#2590=EDGE_CURVE ( 'NONE', #3533, #5822, #7418, .T. ) ;
#2596=DIRECTION ( 'NONE',  ( 1.000000000000000000, 0.000000000000000000, 0.000000000000000000 ) ) ;
#2604=VERTEX_POINT ( 'NONE', #4380 ) ;
#2608=DIRECTION ( 'NONE',  ( 0.000000000000000000, -0.000000000000000000, -1.000000000000000000 ) ) ;
#2620=DIRECTION ( 'NONE',  ( -0.000000000000000000, -0.000000000000000000, 1.000000000000000000 ) ) ;
#2625=FACE_BOUND ( 'NONE', #5111, .T. ) ;
#2627=FACE_OUTER_BOUND ( 'NONE', #5032, .T. ) ;
#2635=VERTEX_POINT ( 'NONE', #6278 ) ;
#2636=ORIENTED_EDGE ( 'NONE', *, *, #138, .T. ) ;
#2638=EDGE_LOOP ( 'NONE', ( #659, #6792, #3594, #963 ) ) ;
#2645=EDGE_CURVE ( 'NONE', #1526, #6086, #1989, .T. ) ;
#2649=ORIENTED_EDGE ( 'NONE', *, *, #2992, .T. ) ;
#2650=DIRECTION ( 'NONE',  ( -0.000000000000000000, -0.000000000000000000, 1.000000000000000000 ) ) ;
#2662=CARTESIAN_POINT ( 'NONE',  ( 0.000000000000000000, 0.000000000000000000, 0.000000000000000000 ) ) ;
#2667=CARTESIAN_POINT ( 'NONE',  ( 89.90381056766652534, -74.99999999999882050, 0.000000000000000000 ) ) ;
#2687=EDGE_CURVE ( 'NONE', #4189, #6783, #4126, .T. ) ;
#2694=ADVANCED_FACE ( 'NONE', ( #1690 ), #7089, .T. ) ;
#2701=AXIS2_PLACEMENT_3D ( 'NONE', #6370, #5261, #2740 ) ;
#2722=ORIENTED_EDGE ( 'NONE', *, *, #5103, .T. ) ;
#2724=( NAMED_UNIT ( * ) SI_UNIT ( $, .STERADIAN. ) SOLID_ANGLE_UNIT ( ) );
#2740=DIRECTION ( 'NONE',  ( -1.000000000000000000, 0.000000000000000000, 0.000000000000000000 ) ) ;
#2750=EDGE_CURVE ( 'NONE', #1651, #5807, #2957, .T. ) ;
#2763=ORIENTED_EDGE ( 'NONE', *, *, #3423, .T. ) ;
#2764=DIRECTION ( 'NONE',  ( -0.000000000000000000, -0.000000000000000000, 1.000000000000000000 ) ) ;
#2766=CYLINDRICAL_SURFACE ( 'NONE', #2455, 30.00000000000000000 ) ;
#2770=VECTOR ( 'NONE', #2374, 1000.000000000000000 ) ;
#2772=CARTESIAN_POINT ( 'NONE',  ( 26.26644452187053957, 80.83980388508807380, 0.000000000000000000 ) ) ;
#2780=ADVANCED_FACE ( 'NONE', ( #2874 ), #1210, .T. ) ;
#2787=CARTESIAN_POINT ( 'NONE',  ( -74.01644452187024115, -49.96174644486060856, 10.00000000000000000 ) ) ;
#2791=ORIENTED_EDGE ( 'NONE', *, *, #1375, .F. ) ;
#2803=LINE ( 'NONE', #5202, #6564 ) ;
#2814=FACE_OUTER_BOUND ( 'NONE', #4238, .T. ) ;
#2815=ORIENTED_EDGE ( 'NONE', *, *, #7459, .T. ) ;
#2824=CIRCLE ( 'NONE', #5468, 30.00000000000000000 ) ;
#2838=EDGE_CURVE ( 'NONE', #3509, #5165, #7209, .T. ) ;
#2848=EDGE_CURVE ( 'NONE', #7033, #6826, #1812, .T. ) ;
#2851=AXIS2_PLACEMENT_3D ( 'NONE', #6290, #955, #175 ) ;
#2853=CYLINDRICAL_SURFACE ( 'NONE', #1926, 5.249999999999997335 ) ;
#2858=CARTESIAN_POINT ( 'NONE',  ( 0.000000000000000000, 0.000000000000000000, 10.00000000000000000 ) ) ;
#2860=DIRECTION ( 'NONE',  ( 1.000000000000000000, 0.000000000000000000, 0.000000000000000000 ) ) ;
#2865=VERTEX_POINT ( 'NONE', #5870 ) ;
#2874=FACE_OUTER_BOUND ( 'NONE', #755, .T. ) ;
#2887=DIRECTION ( 'NONE',  ( -0.000000000000000000, -0.000000000000000000, 1.000000000000000000 ) ) ;
#2896=ORIENTED_EDGE ( 'NONE', *, *, #3134, .F. ) ;
#2915=DIRECTION ( 'NONE',  ( -0.000000000000000000, -0.000000000000000000, 1.000000000000000000 ) ) ;
#2916=ORIENTED_EDGE ( 'NONE', *, *, #2927, .T. ) ;
#2923=DIRECTION ( 'NONE',  ( -0.000000000000000000, -0.000000000000000000, 1.000000000000000000 ) ) ;
#2925=VERTEX_POINT ( 'NONE', #6144 ) ;
#2927=EDGE_CURVE ( 'NONE', #1526, #4732, #5655, .T. ) ;
#2934=AXIS2_PLACEMENT_3D ( 'NONE', #437, #5255, #2269 ) ;
#2941=DIRECTION ( 'NONE',  ( 0.000000000000000000, 0.000000000000000000, 1.000000000000000000 ) ) ;
#2944=FACE_BOUND ( 'NONE', #1861, .T. ) ;
#2948=APPLICATION_CONTEXT ( 'automotive_design' ) ;
#2949=ORIENTED_EDGE ( 'NONE', *, *, #6385, .T. ) ;
#2955=VECTOR ( 'NONE', #2923, 1000.000000000000000 ) ;
#2957=LINE ( 'NONE', #4089, #1628 ) ;
#2963=CARTESIAN_POINT ( 'NONE',  ( -10.00000000000000000, 0.000000000000000000, 0.000000000000000000 ) ) ;
#2970=DIRECTION ( 'NONE',  ( -1.000000000000000000, 0.000000000000000000, 0.000000000000000000 ) ) ;
#2981=FACE_BOUND ( 'NONE', #848, .T. ) ;
#2992=EDGE_CURVE ( 'NONE', #3509, #924, #6419, .T. ) ;
#2995=DIRECTION ( 'NONE',  ( 0.000000000000000000, 0.000000000000000000, -1.000000000000000000 ) ) ;
#3035=( NAMED_UNIT ( * ) PLANE_ANGLE_UNIT ( ) SI_UNIT ( $, .RADIAN. ) );
#3038=CIRCLE ( 'NONE', #7430, 5.250000000000000888 ) ;
#3042=ORIENTED_EDGE ( 'NONE', *, *, #5245, .T. ) ;
#3049=CIRCLE ( 'NONE', #7442, 5.250000000000004441 ) ;
#3058=DIRECTION ( 'NONE',  ( 1.000000000000000000, 0.000000000000000000, 0.000000000000000000 ) ) ;
#3073=EDGE_CURVE ( 'NONE', #5822, #7440, #5790, .T. ) ;
#3082=AXIS2_PLACEMENT_3D ( 'NONE', #2055, #2608, #969 ) ;
#3084=AXIS2_PLACEMENT_3D ( 'NONE', #2772, #1544, #1467 ) ;
#3092=ORIENTED_EDGE ( 'NONE', *, *, #5346, .F. ) ;
#3100=DIRECTION ( 'NONE',  ( -0.000000000000000000, -0.000000000000000000, 1.000000000000000000 ) ) ;
#3126=AXIS2_PLACEMENT_3D ( 'NONE', #6016, #7315, #4308 ) ;
#3133=AXIS2_PLACEMENT_3D ( 'NONE', #402, #7119, #1717 ) ;
#3134=EDGE_CURVE ( 'NONE', #5121, #7260, #3648, .T. ) ;
#3139=CARTESIAN_POINT ( 'NONE',  ( 31.51644452187053602, 80.83980388508807380, 0.000000000000000000 ) ) ;
#3151=CARTESIAN_POINT ( 'NONE',  ( 0.000000000000000000, 0.000000000000000000, 10.00000000000000000 ) ) ;
#3152=DIRECTION ( 'NONE',  ( 1.000000000000000000, 0.000000000000000000, 0.000000000000000000 ) ) ;
#3161=DIRECTION ( 'NONE',  ( -0.000000000000000000, 1.000000000000000000, 0.000000000000000000 ) ) ;
#3166=FACE_OUTER_BOUND ( 'NONE', #8, .T. ) ;
#3167=SURFACE_SIDE_STYLE ('',( #161 ) ) ;
#3173=EDGE_CURVE ( 'NONE', #5558, #5183, #740, .T. ) ;
#3184=DIRECTION ( 'NONE',  ( 0.000000000000000000, 0.000000000000000000, 1.000000000000000000 ) ) ;
#3186=DIRECTION ( 'NONE',  ( -0.000000000000000000, -0.000000000000000000, 1.000000000000000000 ) ) ;
#3187=PLANE ( 'NONE',  #5387 ) ;
#3190=ORIENTED_EDGE ( 'NONE', *, *, #6553, .F. ) ;
#3200=ORIENTED_EDGE ( 'NONE', *, *, #82, .F. ) ;
#3201=CARTESIAN_POINT ( 'NONE',  ( 26.26644452187122170, -80.83980388508783221, 0.000000000000000000 ) ) ;
#3207=EDGE_CURVE ( 'NONE', #2604, #7338, #4368, .T. ) ;
#3236=CARTESIAN_POINT ( 'NONE',  ( 89.90381056766652534, -74.99999999999882050, 10.00000000000000000 ) ) ;
#3238=ORIENTED_EDGE ( 'NONE', *, *, #7448, .F. ) ;
#3240=EDGE_LOOP ( 'NONE', ( #853, #5036, #2416, #2452, #4343, #2949, #5078, #7734, #1440, #2916, #33, #5444, #3482, #4229, #255 ) ) ;
#3256=DIRECTION ( 'NONE',  ( 0.000000000000000000, 0.000000000000000000, -1.000000000000000000 ) ) ;
#3263=ORIENTED_EDGE ( 'NONE', *, *, #6406, .T. ) ;
#3264=EDGE_CURVE ( 'NONE', #6807, #5454, #7444, .T. ) ;
#3287=CYLINDRICAL_SURFACE ( 'NONE', #6730, 150.0000000000000568 ) ;
#3290=VERTEX_POINT ( 'NONE', #4526 ) ;
#3309=EDGE_CURVE ( 'NONE', #294, #989, #2172, .T. ) ;
#3315=FACE_OUTER_BOUND ( 'NONE', #6561, .T. ) ;
#3325=CARTESIAN_POINT ( 'NONE',  ( 129.9038105676665396, -74.99999999999882050, 0.000000000000000000 ) ) ;
#3328=CIRCLE ( 'NONE', #1822, 40.00000000000000711 ) ;
#3330=DIRECTION ( 'NONE',  ( 0.000000000000000000, 0.000000000000000000, 1.000000000000000000 ) ) ;
#3352=ORIENTED_EDGE ( 'NONE', *, *, #7040, .T. ) ;
#3353=CARTESIAN_POINT ( 'NONE',  ( -68.76644452187068168, 49.96174644486002592, 0.000000000000000000 ) ) ;
#3356=CARTESIAN_POINT ( 'NONE',  ( -39.64284999284934941, 144.6666666666667140, 5.000000000000000000 ) ) ;
#3364=CARTESIAN_POINT ( 'NONE',  ( 10.00000000000000000, 28.28427124746190202, 0.000000000000000000 ) ) ;
#3368=EDGE_CURVE ( 'NONE', #5511, #2491, #5038, .T. ) ;
#3374=CARTESIAN_POINT ( 'NONE',  ( -145.1064334105733451, -38.00161816111073421, 0.000000000000000000 ) ) ;
#3376=CARTESIAN_POINT ( 'NONE',  ( -10.00000000000000000, 42.00000000000000000, 0.000000000000000000 ) ) ;
#3378=VERTEX_POINT ( 'NONE', #7028 ) ;
#3381=CARTESIAN_POINT ( 'NONE',  ( 10.00000000000000000, 28.28427124746190202, 10.00000000000000000 ) ) ;
#3382=CARTESIAN_POINT ( 'NONE',  ( 39.64284999284934230, -144.6666666666667140, 0.000000000000000000 ) ) ;
#3387=VECTOR ( 'NONE', #4419, 1000.000000000000000 ) ;
#3388=CARTESIAN_POINT ( 'NONE',  ( 31.51644452187122525, -80.83980388508783221, 10.00000000000000000 ) ) ;
#3391=VERTEX_POINT ( 'NONE', #2386 ) ;
#3396=CARTESIAN_POINT ( 'NONE',  ( 0.000000000000000000, 0.000000000000000000, 0.000000000000000000 ) ) ;
#3399=DIRECTION ( 'NONE',  ( 0.000000000000000000, 0.000000000000000000, 1.000000000000000000 ) ) ;
#3401=LINE ( 'NONE', #7189, #7030 ) ;
#3423=EDGE_CURVE ( 'NONE', #589, #3903, #5841, .T. ) ;
#3427=CARTESIAN_POINT ( 'NONE',  ( 79.75000000000000000, 9.726431976288768917E-13, 10.00000000000000000 ) ) ;
#3428=CIRCLE ( 'NONE', #4182, 150.0000000000000568 ) ;
#3454=ORIENTED_EDGE ( 'NONE', *, *, #6025, .F. ) ;
#3463=DIRECTION ( 'NONE',  ( -0.000000000000000000, -0.000000000000000000, 1.000000000000000000 ) ) ;
#3473=CARTESIAN_POINT ( 'NONE',  ( 21.01644452187122170, -80.83980388508783221, 10.00000000000000000 ) ) ;
#3482=ORIENTED_EDGE ( 'NONE', *, *, #938, .T. ) ;
#3484=AXIS2_PLACEMENT_3D ( 'NONE', #1065, #6361, #1662 ) ;
#3497=EDGE_CURVE ( 'NONE', #2604, #6348, #3535, .T. ) ;
#3502=DIRECTION ( 'NONE',  ( -1.000000000000000000, 0.000000000000000000, 0.000000000000000000 ) ) ;
#3509=VERTEX_POINT ( 'NONE', #7614 ) ;
#3511=CARTESIAN_POINT ( 'NONE',  ( 129.9038105676649764, 75.00000000000153477, 0.000000000000000000 ) ) ;
#3512=DIRECTION ( 'NONE',  ( -0.000000000000000000, -0.000000000000000000, 1.000000000000000000 ) ) ;
#3518=DIRECTION ( 'NONE',  ( 0.000000000000000000, 0.000000000000000000, 1.000000000000000000 ) ) ;
#3519=DIRECTION ( 'NONE',  ( -0.000000000000000000, 1.000000000000000000, 0.000000000000000000 ) ) ;
#3525=DIRECTION ( 'NONE',  ( 1.000000000000000000, 0.000000000000000000, 0.000000000000000000 ) ) ;
#3527=( LENGTH_UNIT ( ) NAMED_UNIT ( * ) SI_UNIT ( .MILLI., .METRE. ) );
#3528=FACE_BOUND ( 'NONE', #3819, .T. ) ;
#3532=PRODUCT_DEFINITION_CONTEXT ( 'detailed design', #2948, 'design' ) ;
#3533=VERTEX_POINT ( 'NONE', #784 ) ;
#3534=ORIENTED_EDGE ( 'NONE', *, *, #314, .F. ) ;
#3535=CIRCLE ( 'NONE', #6310, 40.00000000000000000 ) ;
#3555=CARTESIAN_POINT ( 'NONE',  ( 0.000000000000000000, 0.000000000000000000, 10.00000000000000000 ) ) ;
#3559=CIRCLE ( 'NONE', #6840, 40.00000000000000711 ) ;
#3562=ORIENTED_EDGE ( 'NONE', *, *, #754, .F. ) ;
#3578=DIRECTION ( 'NONE',  ( -1.000000000000000000, 0.000000000000000000, 0.000000000000000000 ) ) ;
#3584=VECTOR ( 'NONE', #3972, 1000.000000000000000 ) ;
#3585=MECHANICAL_DESIGN_GEOMETRIC_PRESENTATION_REPRESENTATION('',(#6481),#1829);
#3590=PRODUCT_DEFINITION ( 'UNKNOWN', '', #38, #3532 ) ;
#3593=PRODUCT_DEFINITION_SHAPE ( 'NONE', 'NONE',  #3590 ) ;
#3594=ORIENTED_EDGE ( 'NONE', *, *, #3713, .F. ) ;
#3600=DIRECTION ( 'NONE',  ( -0.000000000000000000, -0.000000000000000000, 1.000000000000000000 ) ) ;
#3604=ADVANCED_FACE ( 'NONE', ( #3166 ), #5522, .F. ) ;
#3605=ORIENTED_EDGE ( 'NONE', *, *, #6346, .F. ) ;
#3607=ORIENTED_EDGE ( 'NONE', *, *, #3173, .T. ) ;
#3608=AXIS2_PLACEMENT_3D ( 'NONE', #1241, #5464, #6921 ) ;
#3616=CIRCLE ( 'NONE', #3484, 40.00000000000000711 ) ;
#3624=CARTESIAN_POINT ( 'NONE',  ( -150.0000000000000568, 0.000000000000000000, 10.00000000000000000 ) ) ;
#3640=ORIENTED_EDGE ( 'NONE', *, *, #3895, .T. ) ;
#3648=CIRCLE ( 'NONE', #2152, 5.249999999999997335 ) ;
#3651=ORIENTED_EDGE ( 'NONE', *, *, #3207, .T. ) ;
#3653=EDGE_CURVE ( 'NONE', #7033, #6563, #7313, .T. ) ;
#3678=ORIENTED_EDGE ( 'NONE', *, *, #795, .T. ) ;
#3698=EDGE_CURVE ( 'NONE', #3533, #2245, #5927, .T. ) ;
#3702=EDGE_CURVE ( 'NONE', #6571, #7478, #6430, .T. ) ;
#3708=EDGE_CURVE ( 'NONE', #5120, #3378, #3038, .T. ) ;
#3713=EDGE_CURVE ( 'NONE', #4996, #4712, #760, .T. ) ;
#3724=DIRECTION ( 'NONE',  ( -0.000000000000000000, -0.000000000000000000, 1.000000000000000000 ) ) ;
#3730=LINE ( 'NONE', #5428, #1143 ) ;
#3754=ORIENTED_EDGE ( 'NONE', *, *, #3134, .T. ) ;
#3758=DIRECTION ( 'NONE',  ( 0.000000000000000000, 0.000000000000000000, 1.000000000000000000 ) ) ;
#3760=CARTESIAN_POINT ( 'NONE',  ( -30.00000000000000000, 3.673940397442059178E-15, 0.000000000000000000 ) ) ;
#3769=ORIENTED_EDGE ( 'NONE', *, *, #2012, .F. ) ;
#3772=AXIS2_PLACEMENT_3D ( 'NONE', #5936, #1911, #3058 ) ;
#3778=EDGE_LOOP ( 'NONE', ( #2526, #3042, #307, #1019 ) ) ;
#3807=ADVANCED_FACE ( 'NONE', ( #3315 ), #4612, .F. ) ;
#3811=VECTOR ( 'NONE', #6248, 1000.000000000000000 ) ;
#3816=DIRECTION ( 'NONE',  ( 0.000000000000000000, 0.000000000000000000, 1.000000000000000000 ) ) ;
#3819=EDGE_LOOP ( 'NONE', ( #4753, #1070 ) ) ;
#3820=ORIENTED_EDGE ( 'NONE', *, *, #5128, .F. ) ;
#3821=ORIENTED_EDGE ( 'NONE', *, *, #508, .T. ) ;
#3825=CARTESIAN_POINT ( 'NONE',  ( -10.00000000000000000, 28.28427124746190202, 0.000000000000000000 ) ) ;
#3829=DIRECTION ( 'NONE',  ( 1.000000000000000000, 0.000000000000000000, 0.000000000000000000 ) ) ;
#3831=CARTESIAN_POINT ( 'NONE',  ( -74.01644452187068168, 49.96174644486002592, 10.00000000000000000 ) ) ;
#3842=EDGE_CURVE ( 'NONE', #7033, #7338, #2290, .T. ) ;
#3843=LINE ( 'NONE', #3880, #2180 ) ;
#3852=AXIS2_PLACEMENT_3D ( 'NONE', #5353, #7632, #5268 ) ;
#3876=CARTESIAN_POINT ( 'NONE',  ( 145.1064334105738567, -38.00161816110871627, 5.000000000000000000 ) ) ;
#3880=CARTESIAN_POINT ( 'NONE',  ( 145.1064334105730893, 38.00161816111175739, 5.000000000000000000 ) ) ;
#3882=CARTESIAN_POINT ( 'NONE',  ( 0.000000000000000000, 0.000000000000000000, 10.00000000000000000 ) ) ;
#3885=FACE_OUTER_BOUND ( 'NONE', #5707, .T. ) ;
#3895=EDGE_CURVE ( 'NONE', #4594, #2925, #2803, .T. ) ;
#3902=ORIENTED_EDGE ( 'NONE', *, *, #3895, .F. ) ;
#3903=VERTEX_POINT ( 'NONE', #3427 ) ;
#3904=EDGE_LOOP ( 'NONE', ( #5820, #2285, #1726, #6451 ) ) ;
#3908=PLANE ( 'NONE',  #4899 ) ;
#3912=CARTESIAN_POINT ( 'NONE',  ( -63.51644452187067458, 49.96174644486002592, 10.00000000000000000 ) ) ;
#3917=FACE_BOUND ( 'NONE', #1533, .T. ) ;
#3924=ORIENTED_EDGE ( 'NONE', *, *, #6407, .F. ) ;
#3932=DIRECTION ( 'NONE',  ( 0.000000000000000000, 1.000000000000000000, 0.000000000000000000 ) ) ;
#3934=LINE ( 'NONE', #3236, #1429 ) ;
#3935=ADVANCED_FACE ( 'NONE', ( #6507 ), #7097, .T. ) ;
#3950=ADVANCED_FACE ( 'NONE', ( #110 ), #2530, .T. ) ;
#3972=DIRECTION ( 'NONE',  ( -0.000000000000000000, -0.000000000000000000, 1.000000000000000000 ) ) ;
#3976=AXIS2_PLACEMENT_3D ( 'NONE', #2858, #7622, #3525 ) ;
#3981=DIRECTION ( 'NONE',  ( 1.000000000000000000, 0.000000000000000000, -0.000000000000000000 ) ) ;
#3983=CARTESIAN_POINT ( 'NONE',  ( 0.000000000000000000, 150.0000000000000568, 10.00000000000000000 ) ) ;
#3988=LINE ( 'NONE', #3364, #7235 ) ;
#4009=VECTOR ( 'NONE', #2915, 1000.000000000000000 ) ;
#4016=DIRECTION ( 'NONE',  ( -0.000000000000000000, -0.000000000000000000, 1.000000000000000000 ) ) ;
#4028=CARTESIAN_POINT ( 'NONE',  ( 26.26644452187053957, 80.83980388508807380, 10.00000000000000000 ) ) ;
#4048=ORIENTED_EDGE ( 'NONE', *, *, #4801, .T. ) ;
#4054=CARTESIAN_POINT ( 'NONE',  ( 0.000000000000000000, 0.000000000000000000, 0.000000000000000000 ) ) ;
#4057=ORIENTED_EDGE ( 'NONE', *, *, #5132, .F. ) ;
#4061=DIRECTION ( 'NONE',  ( 0.5000000000000101030, -0.8660254037844328234, 0.000000000000000000 ) ) ;
#4063=AXIS2_PLACEMENT_3D ( 'NONE', #1249, #6071, #3152 ) ;
#4072=EDGE_CURVE ( 'NONE', #589, #4189, #3049, .T. ) ;
#4076=ADVANCED_FACE ( 'NONE', ( #6151 ), #5475, .F. ) ;
#4078=AXIS2_PLACEMENT_3D ( 'NONE', #2252, #5789, #6578 ) ;
#4089=CARTESIAN_POINT ( 'NONE',  ( 105.4635834177251326, -106.6650485055556601, 5.000000000000000000 ) ) ;
#4110=CARTESIAN_POINT ( 'NONE',  ( 129.9038105676665396, -74.99999999999882050, 10.00000000000000000 ) ) ;
#4126=LINE ( 'NONE', #7716, #4009 ) ;
#4129=ORIENTED_EDGE ( 'NONE', *, *, #3264, .F. ) ;
#4132=CIRCLE ( 'NONE', #345, 40.00000000000001421 ) ;
#4136=FACE_OUTER_BOUND ( 'NONE', #6460, .T. ) ;
#4139=EDGE_LOOP ( 'NONE', ( #1760, #450 ) ) ;
#4142=FACE_OUTER_BOUND ( 'NONE', #7224, .T. ) ;
#4146=CARTESIAN_POINT ( 'NONE',  ( 85.00000000000000000, 9.720002580593245511E-13, 10.00000000000000000 ) ) ;
#4148=AXIS2_PLACEMENT_3D ( 'NONE', #2489, #3816, #4876 ) ;
#4168=DIRECTION ( 'NONE',  ( -0.000000000000000000, -0.000000000000000000, -1.000000000000000000 ) ) ;
#4170=ORIENTED_EDGE ( 'NONE', *, *, #7204, .F. ) ;
#4178=DIRECTION ( 'NONE',  ( 1.000000000000000000, 0.000000000000000000, 0.000000000000000000 ) ) ;
#4182=AXIS2_PLACEMENT_3D ( 'NONE', #2662, #1426, #1469 ) ;
#4186=DIRECTION ( 'NONE',  ( -0.000000000000000000, -0.000000000000000000, 1.000000000000000000 ) ) ;
#4187=CARTESIAN_POINT ( 'NONE',  ( 31.51644452187122525, -80.83980388508783221, 10.00000000000000000 ) ) ;
#4189=VERTEX_POINT ( 'NONE', #4447 ) ;
#4196=CARTESIAN_POINT ( 'NONE',  ( 145.1064334105738567, -38.00161816110872337, 0.000000000000000000 ) ) ;
#4201=EDGE_LOOP ( 'NONE', ( #424, #5306, #7023, #2256 ) ) ;
#4209=DIRECTION ( 'NONE',  ( -1.000000000000000000, 0.000000000000000000, 0.000000000000000000 ) ) ;
#4210=ORIENTED_EDGE ( 'NONE', *, *, #5132, .T. ) ;
#4213=ORIENTED_EDGE ( 'NONE', *, *, #6873, .T. ) ;
#4218=ADVANCED_FACE ( 'NONE', ( #7443 ), #6823, .F. ) ;
#4229=ORIENTED_EDGE ( 'NONE', *, *, #6959, .F. ) ;
#4230=AXIS2_PLACEMENT_3D ( 'NONE', #1962, #3184, #6772 ) ;
#4238=EDGE_LOOP ( 'NONE', ( #449, #4213, #4326, #2791 ) ) ;
#4268=CARTESIAN_POINT ( 'NONE',  ( -10.00000000000000000, 0.000000000000000000, 0.000000000000000000 ) ) ;
#4271=EDGE_CURVE ( 'NONE', #924, #4732, #5153, .T. ) ;
#4293=CARTESIAN_POINT ( 'NONE',  ( 129.9038105676665396, -74.99999999999882050, 10.00000000000000000 ) ) ;
#4308=DIRECTION ( 'NONE',  ( 1.000000000000000000, 0.000000000000000000, 0.000000000000000000 ) ) ;
#4316=DIRECTION ( 'NONE',  ( -0.000000000000000000, -0.000000000000000000, 1.000000000000000000 ) ) ;
#4324=DIRECTION ( 'NONE',  ( 1.000000000000000000, 0.000000000000000000, 0.000000000000000000 ) ) ;
#4326=ORIENTED_EDGE ( 'NONE', *, *, #1032, .T. ) ;
#4328=VERTEX_POINT ( 'NONE', #1125 ) ;
#4343=ORIENTED_EDGE ( 'NONE', *, *, #3713, .T. ) ;
#4349=DIRECTION ( 'NONE',  ( 1.000000000000000000, 0.000000000000000000, 0.000000000000000000 ) ) ;
#4352=ORIENTED_EDGE ( 'NONE', *, *, #529, .F. ) ;
#4354=CARTESIAN_POINT ( 'NONE',  ( -68.76644452187068168, 49.96174644486002592, 10.00000000000000000 ) ) ;
#4367=CARTESIAN_POINT ( 'NONE',  ( -145.1064334105733451, -38.00161816111073421, 5.000000000000000000 ) ) ;
#4368=LINE ( 'NONE', #6785, #1129 ) ;
#4372=EDGE_LOOP ( 'NONE', ( #797, #5509, #4609, #7477 ) ) ;
#4380=CARTESIAN_POINT ( 'NONE',  ( 89.90381056766497636, 75.00000000000153477, 10.00000000000000000 ) ) ;
#4386=CYLINDRICAL_SURFACE ( 'NONE', #1695, 5.250000000000004441 ) ;
#4393=FACE_OUTER_BOUND ( 'NONE', #2569, .T. ) ;
#4396=FACE_OUTER_BOUND ( 'NONE', #6170, .T. ) ;
#4397=CARTESIAN_POINT ( 'NONE',  ( -74.01644452187068168, 49.96174644486002592, 10.00000000000000000 ) ) ;
#4398=DIRECTION ( 'NONE',  ( 0.000000000000000000, 0.000000000000000000, 1.000000000000000000 ) ) ;
#4404=ORIENTED_EDGE ( 'NONE', *, *, #5128, .T. ) ;
#4406=DIRECTION ( 'NONE',  ( 0.000000000000000000, 0.000000000000000000, -1.000000000000000000 ) ) ;
#4409=DIRECTION ( 'NONE',  ( 1.000000000000000000, 0.000000000000000000, 0.000000000000000000 ) ) ;
#4414=AXIS2_PLACEMENT_3D ( 'NONE', #43, #2467, #1942 ) ;
#4419=DIRECTION ( 'NONE',  ( -0.000000000000000000, -0.000000000000000000, 1.000000000000000000 ) ) ;
#4422=ORIENTED_EDGE ( 'NONE', *, *, #7121, .F. ) ;
#4434=CIRCLE ( 'NONE', #1024, 5.250000000000004441 ) ;
#4443=VECTOR ( 'NONE', #2887, 1000.000000000000000 ) ;
#4447=CARTESIAN_POINT ( 'NONE',  ( 90.25000000000001421, 9.720002580593245511E-13, 0.000000000000000000 ) ) ;
#4452=VERTEX_POINT ( 'NONE', #580 ) ;
#4456=( NAMED_UNIT ( * ) PLANE_ANGLE_UNIT ( ) SI_UNIT ( $, .RADIAN. ) );
#4469=EDGE_CURVE ( 'NONE', #2865, #4328, #7660, .T. ) ;
#4472=FACE_OUTER_BOUND ( 'NONE', #6893, .T. ) ;
#4491=ORIENTED_EDGE ( 'NONE', *, *, #6873, .F. ) ;
#4502=CARTESIAN_POINT ( 'NONE',  ( 0.000000000000000000, -150.0000000000000568, 0.000000000000000000 ) ) ;
#4506=EDGE_LOOP ( 'NONE', ( #1149, #3651, #4544, #1403 ) ) ;
#4514=CARTESIAN_POINT ( 'NONE',  ( 26.26644452187122170, -80.83980388508783221, 10.00000000000000000 ) ) ;
#4522=CIRCLE ( 'NONE', #5139, 30.00000000000000000 ) ;
#4526=CARTESIAN_POINT ( 'NONE',  ( 89.90381056766652534, -74.99999999999882050, 10.00000000000000000 ) ) ;
#4534=DIRECTION ( 'NONE',  ( 0.000000000000000000, 0.000000000000000000, 1.000000000000000000 ) ) ;
#4535=DIRECTION ( 'NONE',  ( 1.000000000000000000, 0.000000000000000000, 0.000000000000000000 ) ) ;
#4544=ORIENTED_EDGE ( 'NONE', *, *, #3842, .F. ) ;
#4559=EDGE_CURVE ( 'NONE', #2491, #5454, #5429, .T. ) ;
#4566=CIRCLE ( 'NONE', #665, 150.0000000000000568 ) ;
#4579=DIRECTION ( 'NONE',  ( 0.000000000000000000, 0.000000000000000000, -1.000000000000000000 ) ) ;
#4589=DIRECTION ( 'NONE',  ( -0.000000000000000000, -0.000000000000000000, 1.000000000000000000 ) ) ;
#4594=VERTEX_POINT ( 'NONE', #5105 ) ;
#4596=ORIENTED_EDGE ( 'NONE', *, *, #3309, .F. ) ;
#4600=ADVANCED_FACE ( 'NONE', ( #6886 ), #7505, .F. ) ;
#4609=ORIENTED_EDGE ( 'NONE', *, *, #6407, .T. ) ;
#4611=ORIENTED_EDGE ( 'NONE', *, *, #7040, .F. ) ;
#4612=CYLINDRICAL_SURFACE ( 'NONE', #5552, 5.249999999999997335 ) ;
#4613=EDGE_CURVE ( 'NONE', #7150, #699, #5585, .T. ) ;
#4618=CARTESIAN_POINT ( 'NONE',  ( 0.000000000000000000, 0.000000000000000000, 0.000000000000000000 ) ) ;
#4647=CIRCLE ( 'NONE', #3772, 40.00000000000000711 ) ;
#4651=LINE ( 'NONE', #3473, #2955 ) ;
#4658=CARTESIAN_POINT ( 'NONE',  ( 0.000000000000000000, 0.000000000000000000, 0.000000000000000000 ) ) ;
#4661=AXIS2_PLACEMENT_3D ( 'NONE', #7379, #1986, #6196 ) ;
#4662=CARTESIAN_POINT ( 'NONE',  ( 39.64284999284935651, 144.6666666666667140, 0.000000000000000000 ) ) ;
#4663=EDGE_LOOP ( 'NONE', ( #7032, #3238, #6513, #5899 ) ) ;
#4667=CARTESIAN_POINT ( 'NONE',  ( 0.000000000000000000, 0.000000000000000000, 0.000000000000000000 ) ) ;
#4668=DIRECTION ( 'NONE',  ( 0.000000000000000000, 0.000000000000000000, 1.000000000000000000 ) ) ;
#4680=DIRECTION ( 'NONE',  ( 0.000000000000000000, -0.000000000000000000, -1.000000000000000000 ) ) ;
#4685=DIRECTION ( 'NONE',  ( 1.000000000000000000, 0.000000000000000000, 0.000000000000000000 ) ) ;
#4690=ORIENTED_EDGE ( 'NONE', *, *, #1278, .F. ) ;
#4696=DIRECTION ( 'NONE',  ( 0.000000000000000000, 0.000000000000000000, 1.000000000000000000 ) ) ;
#4701=ORIENTED_EDGE ( 'NONE', *, *, #314, .T. ) ;
#4703=AXIS2_PLACEMENT_3D ( 'NONE', #976, #6393, #4535 ) ;
#4708=ADVANCED_FACE ( 'NONE', ( #1434 ), #6254, .F. ) ;
#4709=DIRECTION ( 'NONE',  ( 1.000000000000000000, 0.000000000000000000, 0.000000000000000000 ) ) ;
#4712=VERTEX_POINT ( 'NONE', #2667 ) ;
#4717=CIRCLE ( 'NONE', #1828, 30.00000000000000000 ) ;
#4727=ORIENTED_EDGE ( 'NONE', *, *, #6970, .T. ) ;
#4728=DIRECTION ( 'NONE',  ( 0.000000000000000000, 0.000000000000000000, 1.000000000000000000 ) ) ;
#4731=CIRCLE ( 'NONE', #3852, 5.250000000000004441 ) ;
#4732=VERTEX_POINT ( 'NONE', #3374 ) ;
#4749=AXIS2_PLACEMENT_3D ( 'NONE', #6498, #2995, #3578 ) ;
#4753=ORIENTED_EDGE ( 'NONE', *, *, #82, .T. ) ;
#4754=ADVANCED_FACE ( 'NONE', ( #5178 ), #2322, .F. ) ;
#4766=ORIENTED_EDGE ( 'NONE', *, *, #223, .F. ) ;
#4769=DIRECTION ( 'NONE',  ( 0.5000000000000101030, -0.8660254037844328234, 0.000000000000000000 ) ) ;
#4776=DIRECTION ( 'NONE',  ( 0.000000000000000000, 0.000000000000000000, 1.000000000000000000 ) ) ;
#4780=VECTOR ( 'NONE', #3463, 1000.000000000000000 ) ;
#4784=CARTESIAN_POINT ( 'NONE',  ( 79.75000000000000000, 9.726431976288768917E-13, 0.000000000000000000 ) ) ;
#4798=AXIS2_PLACEMENT_3D ( 'NONE', #1292, #1215, #590 ) ;
#4801=EDGE_CURVE ( 'NONE', #3903, #6783, #114, .T. ) ;
#4803=ADVANCED_FACE ( 'NONE', ( #5892 ), #6999, .F. ) ;
#4814=CYLINDRICAL_SURFACE ( 'NONE', #1233, 5.250000000000004441 ) ;
#4815=CARTESIAN_POINT ( 'NONE',  ( -63.51644452187023404, -49.96174644486060856, 10.00000000000000000 ) ) ;
#4823=CARTESIAN_POINT ( 'NONE',  ( 21.01644452187054313, 80.83980388508807380, 0.000000000000000000 ) ) ;
#4830=FACE_OUTER_BOUND ( 'NONE', #1682, .T. ) ;
#4835=CARTESIAN_POINT ( 'NONE',  ( 105.4635834177251326, -106.6650485055556601, 0.000000000000000000 ) ) ;
#4836=DIRECTION ( 'NONE',  ( -0.000000000000000000, -0.000000000000000000, -1.000000000000000000 ) ) ;
#4840=VECTOR ( 'NONE', #5304, 1000.000000000000000 ) ;
#4872=DIRECTION ( 'NONE',  ( 1.000000000000000000, 0.000000000000000000, 0.000000000000000000 ) ) ;
#4876=DIRECTION ( 'NONE',  ( -0.5000000000000037748, 0.8660254037844364872, 0.000000000000000000 ) ) ;
#4878=ORIENTED_EDGE ( 'NONE', *, *, #4271, .T. ) ;
#4891=( NAMED_UNIT ( * ) PLANE_ANGLE_UNIT ( ) SI_UNIT ( $, .RADIAN. ) );
#4895=CARTESIAN_POINT ( 'NONE',  ( 31.51644452187053602, 80.83980388508807380, 10.00000000000000000 ) ) ;
#4899=AXIS2_PLACEMENT_3D ( 'NONE', #6277, #2145, #3981 ) ;
#4908=DIRECTION ( 'NONE',  ( 1.000000000000000000, 0.000000000000000000, 0.000000000000000000 ) ) ;
#4919=VERTEX_POINT ( 'NONE', #6055 ) ;
#4939=CARTESIAN_POINT ( 'NONE',  ( 0.000000000000000000, 0.000000000000000000, 10.00000000000000000 ) ) ;
#4956=ORIENTED_EDGE ( 'NONE', *, *, #4559, .F. ) ;
#4968=CIRCLE ( 'NONE', #1430, 40.00000000000000711 ) ;
#4972=COLOUR_RGB ( '',0.8941176470588234615, 0.8941176470588234615, 0.8941176470588234615 ) ;
#4996=VERTEX_POINT ( 'NONE', #4196 ) ;
#4999=CIRCLE ( 'NONE', #6642, 5.249999999999997335 ) ;
#5000=EDGE_CURVE ( 'NONE', #1572, #5558, #7174, .T. ) ;
#5004=EDGE_CURVE ( 'NONE', #1194, #6563, #4647, .T. ) ;
#5009=DIRECTION ( 'NONE',  ( 1.000000000000000000, 0.000000000000000000, 0.000000000000000000 ) ) ;
#5010=SHAPE_REPRESENTATION_RELATIONSHIP ( 'NONE' , 'NONE' ,  #637, #5187 ) ;
#5022=CARTESIAN_POINT ( 'NONE',  ( 145.1064334105738567, -38.00161816110870916, 10.00000000000000000 ) ) ;
#5024=AXIS2_PLACEMENT_3D ( 'NONE', #6647, #570, #1234 ) ;
#5029=CARTESIAN_POINT ( 'NONE',  ( 105.4635834177251326, -106.6650485055556601, 10.00000000000000000 ) ) ;
#5030=DIRECTION ( 'NONE',  ( 1.000000000000000000, 0.000000000000000000, 0.000000000000000000 ) ) ;
#5032=EDGE_LOOP ( 'NONE', ( #4878, #1524, #5364, #2059 ) ) ;
#5036=ORIENTED_EDGE ( 'NONE', *, *, #3842, .T. ) ;
#5038=LINE ( 'NONE', #2963, #5922 ) ;
#5041=ADVANCED_FACE ( 'NONE', ( #1115, #3528, #5458, #2944, #2981, #5343, #7741 ), #3908, .F. ) ;
#5046=DIRECTION ( 'NONE',  ( -0.000000000000000000, -0.000000000000000000, 1.000000000000000000 ) ) ;
#5071=ORIENTED_EDGE ( 'NONE', *, *, #6746, .F. ) ;
#5075=AXIS2_PLACEMENT_3D ( 'NONE', #2356, #2941, #5341 ) ;
#5077=ORIENTED_EDGE ( 'NONE', *, *, #4559, .T. ) ;
#5078=ORIENTED_EDGE ( 'NONE', *, *, #138, .F. ) ;
#5103=EDGE_CURVE ( 'NONE', #2925, #57, #4522, .T. ) ;
#5105=CARTESIAN_POINT ( 'NONE',  ( 30.00000000000000000, 0.000000000000000000, 0.000000000000000000 ) ) ;
#5111=EDGE_LOOP ( 'NONE', ( #2439, #1297 ) ) ;
#5114=CIRCLE ( 'NONE', #2106, 150.0000000000000568 ) ;
#5120=VERTEX_POINT ( 'NONE', #6985 ) ;
#5121=VERTEX_POINT ( 'NONE', #3139 ) ;
#5122=CARTESIAN_POINT ( 'NONE',  ( 26.26644452187053957, 80.83980388508807380, 10.00000000000000000 ) ) ;
#5128=EDGE_CURVE ( 'NONE', #3378, #5120, #5590, .T. ) ;
#5132=EDGE_CURVE ( 'NONE', #2245, #7440, #722, .T. ) ;
#5136=EDGE_LOOP ( 'NONE', ( #230, #2763, #4048, #2010 ) ) ;
#5139=AXIS2_PLACEMENT_3D ( 'NONE', #135, #7528, #4349 ) ;
#5153=LINE ( 'NONE', #4367, #5646 ) ;
#5155=LINE ( 'NONE', #3388, #3584 ) ;
#5156=AXIS2_PLACEMENT_3D ( 'NONE', #2299, #3512, #4685 ) ;
#5158=ORIENTED_EDGE ( 'NONE', *, *, #4613, .F. ) ;
#5165=VERTEX_POINT ( 'NONE', #7606 ) ;
#5168=FACE_OUTER_BOUND ( 'NONE', #7736, .T. ) ;
#5177=ADVANCED_FACE ( 'NONE', ( #348 ), #2766, .F. ) ;
#5178=FACE_OUTER_BOUND ( 'NONE', #6855, .T. ) ;
#5183=VERTEX_POINT ( 'NONE', #2301 ) ;
#5187=ADVANCED_BREP_SHAPE_REPRESENTATION ( '', ( #5726, #7485 ), #2086 ) ;
#5202=CARTESIAN_POINT ( 'NONE',  ( 30.00000000000000000, 0.000000000000000000, 0.000000000000000000 ) ) ;
#5203=ADVANCED_FACE ( 'NONE', ( #4136 ), #1060, .F. ) ;
#5215=DIRECTION ( 'NONE',  ( 0.000000000000000000, 0.000000000000000000, 1.000000000000000000 ) ) ;
#5222=CARTESIAN_POINT ( 'NONE',  ( 85.00000000000000000, 9.720002580593245511E-13, 10.00000000000000000 ) ) ;
#5245=EDGE_CURVE ( 'NONE', #5120, #4919, #4651, .T. ) ;
#5251=AXIS2_PLACEMENT_3D ( 'NONE', #6401, #3399, #1704 ) ;
#5255=DIRECTION ( 'NONE',  ( 0.000000000000000000, 0.000000000000000000, 1.000000000000000000 ) ) ;
#5259=DIRECTION ( 'NONE',  ( 0.000000000000000000, 0.000000000000000000, -1.000000000000000000 ) ) ;
#5261=DIRECTION ( 'NONE',  ( -0.000000000000000000, -0.000000000000000000, -1.000000000000000000 ) ) ;
#5266=ORIENTED_EDGE ( 'NONE', *, *, #5245, .F. ) ;
#5268=DIRECTION ( 'NONE',  ( 1.000000000000000000, 0.000000000000000000, 0.000000000000000000 ) ) ;
#5280=DIRECTION ( 'NONE',  ( 1.000000000000000000, 0.000000000000000000, 0.000000000000000000 ) ) ;
#5284=LINE ( 'NONE', #3356, #2567 ) ;
#5298=CARTESIAN_POINT ( 'NONE',  ( 10.00000000000000000, 0.000000000000000000, 10.00000000000000000 ) ) ;
#5299=PRESENTATION_STYLE_ASSIGNMENT (( #5562 ) ) ;
#5300=DIRECTION ( 'NONE',  ( -0.000000000000000000, -0.000000000000000000, 1.000000000000000000 ) ) ;
#5304=DIRECTION ( 'NONE',  ( -0.000000000000000000, -0.000000000000000000, 1.000000000000000000 ) ) ;
#5306=ORIENTED_EDGE ( 'NONE', *, *, #7223, .F. ) ;
#5308=VERTEX_POINT ( 'NONE', #5409 ) ;
#5316=ORIENTED_EDGE ( 'NONE', *, *, #2838, .F. ) ;
#5320=CIRCLE ( 'NONE', #2934, 30.00000000000000000 ) ;
#5341=DIRECTION ( 'NONE',  ( 1.000000000000000000, 0.000000000000000000, 0.000000000000000000 ) ) ;
#5343=FACE_BOUND ( 'NONE', #1925, .T. ) ;
#5346=EDGE_CURVE ( 'NONE', #4452, #3391, #742, .T. ) ;
#5353=CARTESIAN_POINT ( 'NONE',  ( -68.76644452187068168, 49.96174644486002592, 0.000000000000000000 ) ) ;
#5364=ORIENTED_EDGE ( 'NONE', *, *, #2645, .T. ) ;
#5368=ORIENTED_EDGE ( 'NONE', *, *, #4801, .F. ) ;
#5387=AXIS2_PLACEMENT_3D ( 'NONE', #5586, #1886, #2486 ) ;
#5392=AXIS2_PLACEMENT_3D ( 'NONE', #4939, #685, #1349 ) ;
#5409=CARTESIAN_POINT ( 'NONE',  ( 10.00000000000000000, 42.00000000000000000, 10.00000000000000000 ) ) ;
#5412=ORIENTED_EDGE ( 'NONE', *, *, #354, .F. ) ;
#5422=DIRECTION ( 'NONE',  ( -0.4999999999999918954, -0.8660254037844432595, 0.000000000000000000 ) ) ;
#5428=CARTESIAN_POINT ( 'NONE',  ( 0.000000000000000000, 42.00000000000000000, 10.00000000000000000 ) ) ;
#5429=LINE ( 'NONE', #1514, #6536 ) ;
#5444=ORIENTED_EDGE ( 'NONE', *, *, #6878, .F. ) ;
#5447=CIRCLE ( 'NONE', #2056, 30.00000000000000000 ) ;
#5454=VERTEX_POINT ( 'NONE', #6630 ) ;
#5456=DIRECTION ( 'NONE',  ( 1.000000000000000000, 0.000000000000000000, 0.000000000000000000 ) ) ;
#5458=FACE_BOUND ( 'NONE', #4139, .T. ) ;
#5464=DIRECTION ( 'NONE',  ( 0.000000000000000000, 0.000000000000000000, 1.000000000000000000 ) ) ;
#5468=AXIS2_PLACEMENT_3D ( 'NONE', #821, #7560, #4409 ) ;
#5475=CYLINDRICAL_SURFACE ( 'NONE', #889, 40.00000000000000711 ) ;
#5477=EDGE_CURVE ( 'NONE', #699, #294, #3328, .T. ) ;
#5484=ORIENTED_EDGE ( 'NONE', *, *, #3173, .F. ) ;
#5487=CARTESIAN_POINT ( 'NONE',  ( -10.00000000000000000, 42.00000000000000000, 0.000000000000000000 ) ) ;
#5489=CARTESIAN_POINT ( 'NONE',  ( -30.00000000000000000, 3.673940397442059178E-15, 10.00000000000000000 ) ) ;
#5490=ORIENTED_EDGE ( 'NONE', *, *, #2992, .F. ) ;
#5498=ORIENTED_EDGE ( 'NONE', *, *, #3653, .T. ) ;
#5499=VECTOR ( 'NONE', #395, 1000.000000000000000 ) ;
#5509=ORIENTED_EDGE ( 'NONE', *, *, #6297, .T. ) ;
#5511=VERTEX_POINT ( 'NONE', #3825 ) ;
#5521=EDGE_CURVE ( 'NONE', #3378, #6651, #5155, .T. ) ;
#5522=CYLINDRICAL_SURFACE ( 'NONE', #4414, 5.250000000000004441 ) ;
#5523=FILL_AREA_STYLE_COLOUR ( '', #4972 ) ;
#5528=EDGE_CURVE ( 'NONE', #3290, #4712, #3934, .T. ) ;
#5541=ADVANCED_FACE ( 'NONE', ( #1530 ), #1450, .F. ) ;
#5546=CARTESIAN_POINT ( 'NONE',  ( -145.1064334105735725, 38.00161816110971813, 10.00000000000000000 ) ) ;
#5552=AXIS2_PLACEMENT_3D ( 'NONE', #466, #6549, #5914 ) ;
#5558=VERTEX_POINT ( 'NONE', #5635 ) ;
#5559=AXIS2_PLACEMENT_3D ( 'NONE', #24, #1917, #59 ) ;
#5562=SURFACE_STYLE_USAGE ( .BOTH. , #3167 ) ;
#5564=DIRECTION ( 'NONE',  ( -0.5000000000000037748, 0.8660254037844364872, 0.000000000000000000 ) ) ;
#5568=EDGE_CURVE ( 'NONE', #6712, #2925, #2824, .T. ) ;
#5570=PLANE ( 'NONE',  #1417 ) ;
#5575=UNCERTAINTY_MEASURE_WITH_UNIT (LENGTH_MEASURE( 1.000000000000000082E-05 ), #1673, 'distance_accuracy_value', 'NONE');
#5581=PLANE ( 'NONE',  #714 ) ;
#5585=LINE ( 'NONE', #5622, #614 ) ;
#5586=CARTESIAN_POINT ( 'NONE',  ( 10.00000000000000000, 0.000000000000000000, 0.000000000000000000 ) ) ;
#5590=CIRCLE ( 'NONE', #4703, 5.250000000000000888 ) ;
#5592=ORIENTED_EDGE ( 'NONE', *, *, #7459, .F. ) ;
#5613=CARTESIAN_POINT ( 'NONE',  ( -68.76644452187024115, -49.96174644486060856, 10.00000000000000000 ) ) ;
#5622=CARTESIAN_POINT ( 'NONE',  ( 39.64284999284934941, -144.6666666666667140, 5.000000000000000000 ) ) ;
#5627=DIRECTION ( 'NONE',  ( 1.000000000000000000, 0.000000000000000000, 0.000000000000000000 ) ) ;
#5635=CARTESIAN_POINT ( 'NONE',  ( -105.4635834177243794, 106.6650485055563990, 10.00000000000000000 ) ) ;
#5646=VECTOR ( 'NONE', #1366, 1000.000000000000000 ) ;
#5648=CARTESIAN_POINT ( 'NONE',  ( 0.000000000000000000, 0.000000000000000000, 10.00000000000000000 ) ) ;
#5655=CIRCLE ( 'NONE', #4148, 40.00000000000000711 ) ;
#5669=AXIS2_PLACEMENT_3D ( 'NONE', #5122, #5046, #3829 ) ;
#5671=ADVANCED_FACE ( 'NONE', ( #1735 ), #1648, .T. ) ;
#5689=ORIENTED_EDGE ( 'NONE', *, *, #2415, .F. ) ;
#5695=SHAPE_DEFINITION_REPRESENTATION ( #3593, #637 ) ;
#5698=ORIENTED_EDGE ( 'NONE', *, *, #1820, .F. ) ;
#5707=EDGE_LOOP ( 'NONE', ( #5316, #5779, #5689, #6389 ) ) ;
#5711=EDGE_LOOP ( 'NONE', ( #698, #1328, #5158, #2636 ) ) ;
#5726=MANIFOLD_SOLID_BREP ( 'M10 Clearance Hole1', #6748 ) ;
#5727=DIRECTION ( 'NONE',  ( 0.000000000000000000, 0.000000000000000000, 1.000000000000000000 ) ) ;
#5730=CYLINDRICAL_SURFACE ( 'NONE', #959, 5.250000000000004441 ) ;
#5738=ORIENTED_EDGE ( 'NONE', *, *, #2037, .F. ) ;
#5746=DIRECTION ( 'NONE',  ( -0.000000000000000000, -0.000000000000000000, 1.000000000000000000 ) ) ;
#5751=VECTOR ( 'NONE', #5259, 1000.000000000000000 ) ;
#5778=CARTESIAN_POINT ( 'NONE',  ( -30.00000000000000000, 3.673940397442059178E-15, 0.000000000000000000 ) ) ;
#5779=ORIENTED_EDGE ( 'NONE', *, *, #991, .F. ) ;
#5789=DIRECTION ( 'NONE',  ( -0.000000000000000000, -0.000000000000000000, -1.000000000000000000 ) ) ;
#5790=CIRCLE ( 'NONE', #5156, 5.250000000000004441 ) ;
#5791=VERTEX_POINT ( 'NONE', #5546 ) ;
#5798=DIRECTION ( 'NONE',  ( -1.000000000000000000, 0.000000000000000000, 0.000000000000000000 ) ) ;
#5807=VERTEX_POINT ( 'NONE', #4835 ) ;
#5809=LINE ( 'NONE', #364, #5499 ) ;
#5812=EDGE_CURVE ( 'NONE', #6752, #4594, #4717, .T. ) ;
#5820=ORIENTED_EDGE ( 'NONE', *, *, #3423, .F. ) ;
#5822=VERTEX_POINT ( 'NONE', #4397 ) ;
#5830=ORIENTED_EDGE ( 'NONE', *, *, #3207, .F. ) ;
#5841=LINE ( 'NONE', #2231, #1390 ) ;
#5843=CIRCLE ( 'NONE', #3084, 5.249999999999997335 ) ;
#5860=ORIENTED_EDGE ( 'NONE', *, *, #6258, .T. ) ;
#5870=CARTESIAN_POINT ( 'NONE',  ( -74.01644452187024115, -49.96174644486060856, 0.000000000000000000 ) ) ;
#5878=DIRECTION ( 'NONE',  ( -0.000000000000000000, -0.000000000000000000, 1.000000000000000000 ) ) ;
#5881=VECTOR ( 'NONE', #1807, 1000.000000000000000 ) ;
#5892=FACE_OUTER_BOUND ( 'NONE', #5136, .T. ) ;
#5899=ORIENTED_EDGE ( 'NONE', *, *, #5477, .T. ) ;
#5914=DIRECTION ( 'NONE',  ( 1.000000000000000000, 0.000000000000000000, 0.000000000000000000 ) ) ;
#5922=VECTOR ( 'NONE', #3519, 1000.000000000000000 ) ;
#5927=CIRCLE ( 'NONE', #6559, 5.250000000000004441 ) ;
#5929=EDGE_CURVE ( 'NONE', #6752, #6712, #2325, .T. ) ;
#5930=VERTEX_POINT ( 'NONE', #2787 ) ;
#5936=CARTESIAN_POINT ( 'NONE',  ( 0.000000000000000000, 150.0000000000000568, 0.000000000000000000 ) ) ;
#5953=CARTESIAN_POINT ( 'NONE',  ( 0.000000000000000000, 0.000000000000000000, 10.00000000000000000 ) ) ;
#5973=VECTOR ( 'NONE', #3161, 1000.000000000000000 ) ;
#5977=DIRECTION ( 'NONE',  ( 1.000000000000000000, 0.000000000000000000, 0.000000000000000000 ) ) ;
#5979=CARTESIAN_POINT ( 'NONE',  ( 129.9038105676649764, 75.00000000000153477, 10.00000000000000000 ) ) ;
#5981=CARTESIAN_POINT ( 'NONE',  ( -105.4635834177236546, -106.6650485055571380, 10.00000000000000000 ) ) ;
#6014=DIRECTION ( 'NONE',  ( 0.000000000000000000, 0.000000000000000000, 1.000000000000000000 ) ) ;
#6016=CARTESIAN_POINT ( 'NONE',  ( 0.000000000000000000, 150.0000000000000568, 10.00000000000000000 ) ) ;
#6025=EDGE_CURVE ( 'NONE', #2491, #3391, #1598, .T. ) ;
#6030=CARTESIAN_POINT ( 'NONE',  ( 105.4635834177229157, 106.6650485055578912, 5.000000000000000000 ) ) ;
#6050=ORIENTED_EDGE ( 'NONE', *, *, #2590, .F. ) ;
#6055=CARTESIAN_POINT ( 'NONE',  ( 21.01644452187122170, -80.83980388508783221, 10.00000000000000000 ) ) ;
#6067=CARTESIAN_POINT ( 'NONE',  ( -68.76644452187024115, -49.96174644486060856, 10.00000000000000000 ) ) ;
#6069=AXIS2_PLACEMENT_3D ( 'NONE', #2053, #5746, #7517 ) ;
#6071=DIRECTION ( 'NONE',  ( -0.000000000000000000, -0.000000000000000000, 1.000000000000000000 ) ) ;
#6076=DIRECTION ( 'NONE',  ( -0.000000000000000000, -0.000000000000000000, 1.000000000000000000 ) ) ;
#6086=VERTEX_POINT ( 'NONE', #5981 ) ;
#6098=DIRECTION ( 'NONE',  ( -0.000000000000000000, -0.000000000000000000, 1.000000000000000000 ) ) ;
#6133=CARTESIAN_POINT ( 'NONE',  ( 145.1064334105730893, 38.00161816111175739, 0.000000000000000000 ) ) ;
#6138=CARTESIAN_POINT ( 'NONE',  ( 85.00000000000000000, 9.720002580593245511E-13, 10.00000000000000000 ) ) ;
#6144=CARTESIAN_POINT ( 'NONE',  ( 30.00000000000000000, 0.000000000000000000, 10.00000000000000000 ) ) ;
#6150=ORIENTED_EDGE ( 'NONE', *, *, #6959, .T. ) ;
#6151=FACE_OUTER_BOUND ( 'NONE', #6428, .T. ) ;
#6166=CARTESIAN_POINT ( 'NONE',  ( 90.25000000000001421, 9.720002580593245511E-13, 10.00000000000000000 ) ) ;
#6170=EDGE_LOOP ( 'NONE', ( #3821, #6234, #3092, #5592 ) ) ;
#6187=ORIENTED_EDGE ( 'NONE', *, *, #6442, .T. ) ;
#6196=DIRECTION ( 'NONE',  ( 1.000000000000000000, 0.000000000000000000, 0.000000000000000000 ) ) ;
#6198=DIRECTION ( 'NONE',  ( 0.000000000000000000, -0.000000000000000000, 1.000000000000000000 ) ) ;
#6208=UNCERTAINTY_MEASURE_WITH_UNIT (LENGTH_MEASURE( 1.000000000000000082E-05 ), #6695, 'distance_accuracy_value', 'NONE');
#6213=APPLICATION_CONTEXT ( 'automotive_design' ) ;
#6234=ORIENTED_EDGE ( 'NONE', *, *, #795, .F. ) ;
#6240=CARTESIAN_POINT ( 'NONE',  ( -105.4635834177236546, -106.6650485055571380, 5.000000000000000000 ) ) ;
#6242=ORIENTED_EDGE ( 'NONE', *, *, #5000, .T. ) ;
#6248=DIRECTION ( 'NONE',  ( -0.000000000000000000, -0.000000000000000000, 1.000000000000000000 ) ) ;
#6254=CYLINDRICAL_SURFACE ( 'NONE', #6545, 40.00000000000000711 ) ;
#6258=EDGE_CURVE ( 'NONE', #4189, #589, #1157, .T. ) ;
#6277=CARTESIAN_POINT ( 'NONE',  ( 0.000000000000000000, 0.000000000000000000, 0.000000000000000000 ) ) ;
#6278=CARTESIAN_POINT ( 'NONE',  ( 39.64284999284935651, 144.6666666666667140, 10.00000000000000000 ) ) ;
#6280=ORIENTED_EDGE ( 'NONE', *, *, #1531, .F. ) ;
#6290=CARTESIAN_POINT ( 'NONE',  ( -129.9038105676655164, -75.00000000000063949, 10.00000000000000000 ) ) ;
#6297=EDGE_CURVE ( 'NONE', #2865, #5930, #1997, .T. ) ;
#6306=ORIENTED_EDGE ( 'NONE', *, *, #3368, .F. ) ;
#6310=AXIS2_PLACEMENT_3D ( 'NONE', #1663, #4776, #4061 ) ;
#6315=AXIS2_PLACEMENT_3D ( 'NONE', #5953, #1697, #1096 ) ;
#6321=FACE_OUTER_BOUND ( 'NONE', #1275, .T. ) ;
#6332=CARTESIAN_POINT ( 'NONE',  ( -68.76644452187068168, 49.96174644486002592, 10.00000000000000000 ) ) ;
#6336=EDGE_LOOP ( 'NONE', ( #5484, #1825, #510, #6150 ) ) ;
#6340=VERTEX_POINT ( 'NONE', #5022 ) ;
#6346=EDGE_CURVE ( 'NONE', #6348, #2067, #3843, .T. ) ;
#6347=EDGE_LOOP ( 'NONE', ( #5266, #3820, #2282, #1454 ) ) ;
#6348=VERTEX_POINT ( 'NONE', #1508 ) ;
#6349=AXIS2_PLACEMENT_3D ( 'NONE', #1017, #6432, #7099 ) ;
#6356=LINE ( 'NONE', #7648, #4443 ) ;
#6361=DIRECTION ( 'NONE',  ( 0.000000000000000000, 0.000000000000000000, 1.000000000000000000 ) ) ;
#6363=CARTESIAN_POINT ( 'NONE',  ( -63.51644452187067458, 49.96174644486002592, 0.000000000000000000 ) ) ;
#6366=ORIENTED_EDGE ( 'NONE', *, *, #5528, .F. ) ;
#6369=CYLINDRICAL_SURFACE ( 'NONE', #2851, 40.00000000000000711 ) ;
#6370=CARTESIAN_POINT ( 'NONE',  ( 0.000000000000000000, 0.000000000000000000, 10.00000000000000000 ) ) ;
#6385=EDGE_CURVE ( 'NONE', #4712, #5807, #31, .T. ) ;
#6389=ORIENTED_EDGE ( 'NONE', *, *, #6878, .T. ) ;
#6393=DIRECTION ( 'NONE',  ( -0.000000000000000000, -0.000000000000000000, 1.000000000000000000 ) ) ;
#6399=AXIS2_PLACEMENT_3D ( 'NONE', #5979, #4668, #7075 ) ;
#6401=CARTESIAN_POINT ( 'NONE',  ( 0.000000000000000000, 0.000000000000000000, 10.00000000000000000 ) ) ;
#6406=EDGE_CURVE ( 'NONE', #4996, #2067, #3428, .T. ) ;
#6407=EDGE_CURVE ( 'NONE', #5930, #1219, #4434, .T. ) ;
#6419=CIRCLE ( 'NONE', #1503, 150.0000000000000568 ) ;
#6428=EDGE_LOOP ( 'NONE', ( #6366, #624, #1110, #1639 ) ) ;
#6430=CIRCLE ( 'NONE', #5669, 5.249999999999997335 ) ;
#6432=DIRECTION ( 'NONE',  ( 0.000000000000000000, 0.000000000000000000, -1.000000000000000000 ) ) ;
#6440=DIRECTION ( 'NONE',  ( -0.000000000000000000, -0.000000000000000000, 1.000000000000000000 ) ) ;
#6442=EDGE_CURVE ( 'NONE', #4594, #4452, #5447, .T. ) ;
#6451=ORIENTED_EDGE ( 'NONE', *, *, #223, .T. ) ;
#6460=EDGE_LOOP ( 'NONE', ( #3607, #7486, #7012, #4701 ) ) ;
#6461=ORIENTED_EDGE ( 'NONE', *, *, #2838, .T. ) ;
#6463=CIRCLE ( 'NONE', #5075, 30.00000000000000000 ) ;
#6474=VECTOR ( 'NONE', #1422, 1000.000000000000000 ) ;
#6479=ORIENTED_EDGE ( 'NONE', *, *, #5568, .F. ) ;
#6481=STYLED_ITEM ( 'NONE', ( #5299 ), #5187 ) ;
#6482=CARTESIAN_POINT ( 'NONE',  ( -39.64284999284934230, 144.6666666666667140, 0.000000000000000000 ) ) ;
#6498=CARTESIAN_POINT ( 'NONE',  ( 0.000000000000000000, -150.0000000000000568, 10.00000000000000000 ) ) ;
#6500=CIRCLE ( 'NONE', #3976, 150.0000000000000568 ) ;
#6507=FACE_OUTER_BOUND ( 'NONE', #5711, .T. ) ;
#6513=ORIENTED_EDGE ( 'NONE', *, *, #4613, .T. ) ;
#6527=DIRECTION ( 'NONE',  ( 1.000000000000000000, 0.000000000000000000, 0.000000000000000000 ) ) ;
#6536=VECTOR ( 'NONE', #3186, 1000.000000000000000 ) ;
#6545=AXIS2_PLACEMENT_3D ( 'NONE', #7360, #3256, #248 ) ;
#6546=ADVANCED_FACE ( 'NONE', ( #2814 ), #2853, .F. ) ;
#6547=ORIENTED_EDGE ( 'NONE', *, *, #6025, .T. ) ;
#6549=DIRECTION ( 'NONE',  ( -0.000000000000000000, -0.000000000000000000, 1.000000000000000000 ) ) ;
#6553=EDGE_CURVE ( 'NONE', #6807, #6712, #5320, .T. ) ;
#6559=AXIS2_PLACEMENT_3D ( 'NONE', #3353, #2650, #7488 ) ;
#6560=FACE_OUTER_BOUND ( 'NONE', #3904, .T. ) ;
#6561=EDGE_LOOP ( 'NONE', ( #4491, #2896, #6562, #2229 ) ) ;
#6562=ORIENTED_EDGE ( 'NONE', *, *, #1375, .T. ) ;
#6563=VERTEX_POINT ( 'NONE', #4662 ) ;
#6564=VECTOR ( 'NONE', #4016, 1000.000000000000000 ) ;
#6571=VERTEX_POINT ( 'NONE', #4895 ) ;
#6578=DIRECTION ( 'NONE',  ( -1.000000000000000000, 0.000000000000000000, 0.000000000000000000 ) ) ;
#6598=DIRECTION ( 'NONE',  ( 1.000000000000000000, 0.000000000000000000, 0.000000000000000000 ) ) ;
#6603=ORIENTED_EDGE ( 'NONE', *, *, #7121, .T. ) ;
#6605=CIRCLE ( 'NONE', #2580, 150.0000000000000568 ) ;
#6627=ORIENTED_EDGE ( 'NONE', *, *, #7549, .F. ) ;
#6630=CARTESIAN_POINT ( 'NONE',  ( -10.00000000000000000, 42.00000000000000000, 10.00000000000000000 ) ) ;
#6642=AXIS2_PLACEMENT_3D ( 'NONE', #7144, #1145, #2346 ) ;
#6643=EDGE_CURVE ( 'NONE', #4328, #1219, #1304, .T. ) ;
#6647=CARTESIAN_POINT ( 'NONE',  ( 0.000000000000000000, 0.000000000000000000, 10.00000000000000000 ) ) ;
#6651=VERTEX_POINT ( 'NONE', #4187 ) ;
#6662=ORIENTED_EDGE ( 'NONE', *, *, #2037, .T. ) ;
#6665=CARTESIAN_POINT ( 'NONE',  ( 85.00000000000000000, 9.720002580593245511E-13, 0.000000000000000000 ) ) ;
#6676=VECTOR ( 'NONE', #3932, 1000.000000000000000 ) ;
#6695=( LENGTH_UNIT ( ) NAMED_UNIT ( * ) SI_UNIT ( .MILLI., .METRE. ) );
#6697=DIRECTION ( 'NONE',  ( 1.000000000000000000, 0.000000000000000000, 0.000000000000000000 ) ) ;
#6704=CARTESIAN_POINT ( 'NONE',  ( 10.00000000000000000, 0.000000000000000000, 0.000000000000000000 ) ) ;
#6711=CIRCLE ( 'NONE', #1541, 150.0000000000000568 ) ;
#6712=VERTEX_POINT ( 'NONE', #5489 ) ;
#6730=AXIS2_PLACEMENT_3D ( 'NONE', #5648, #240, #7534 ) ;
#6732=ADVANCED_FACE ( 'NONE', ( #6560 ), #1866, .F. ) ;
#6743=DIRECTION ( 'NONE',  ( 0.000000000000000000, 0.000000000000000000, -1.000000000000000000 ) ) ;
#6746=EDGE_CURVE ( 'NONE', #6086, #924, #3559, .T. ) ;
#6748=CLOSED_SHELL ( 'NONE', ( #6546, #2458, #7417, #4600, #4803, #358, #4754, #4708, #5541, #2780, #5671, #7532, #3935, #1038, #7651, #2694, #1137, #5041, #6976, #5203, #460, #1385, #4076, #220, #5177, #1617, #7321, #3950, #6732, #4218, #3604, #1192, #3807 ) ) ;
#6752=VERTEX_POINT ( 'NONE', #3760 ) ;
#6771=DIRECTION ( 'NONE',  ( -0.000000000000000000, -0.000000000000000000, 1.000000000000000000 ) ) ;
#6772=DIRECTION ( 'NONE',  ( 0.4999999999999979461, 0.8660254037844398178, 0.000000000000000000 ) ) ;
#6779=EDGE_LOOP ( 'NONE', ( #4766, #5368 ) ) ;
#6783=VERTEX_POINT ( 'NONE', #6166 ) ;
#6785=CARTESIAN_POINT ( 'NONE',  ( 89.90381056766497636, 75.00000000000153477, 10.00000000000000000 ) ) ;
#6792=ORIENTED_EDGE ( 'NONE', *, *, #5528, .T. ) ;
#6797=AXIS2_PLACEMENT_3D ( 'NONE', #4514, #7432, #2596 ) ;
#6807=VERTEX_POINT ( 'NONE', #6832 ) ;
#6823=CYLINDRICAL_SURFACE ( 'NONE', #6069, 5.250000000000000888 ) ;
#6826=VERTEX_POINT ( 'NONE', #2107 ) ;
#6830=CARTESIAN_POINT ( 'NONE',  ( 129.9038105676665396, -74.99999999999882050, 0.000000000000000000 ) ) ;
#6832=CARTESIAN_POINT ( 'NONE',  ( -9.999999999999998224, 28.28427124746189847, 10.00000000000000000 ) ) ;
#6840=AXIS2_PLACEMENT_3D ( 'NONE', #6869, #271, #5564 ) ;
#6855=EDGE_LOOP ( 'NONE', ( #1600, #3640, #2722, #2815 ) ) ;
#6869=CARTESIAN_POINT ( 'NONE',  ( -129.9038105676655164, -75.00000000000063949, 10.00000000000000000 ) ) ;
#6873=EDGE_CURVE ( 'NONE', #7260, #7478, #6356, .T. ) ;
#6878=EDGE_CURVE ( 'NONE', #2235, #5165, #4566, .T. ) ;
#6886=FACE_OUTER_BOUND ( 'NONE', #3778, .T. ) ;
#6893=EDGE_LOOP ( 'NONE', ( #1041, #6931, #5738, #6242, #3534, #232, #2649, #5071, #3352, #2313, #7639, #1991, #4170, #832, #7280 ) ) ;
#6894=ORIENTED_EDGE ( 'NONE', *, *, #3073, .T. ) ;
#6917=DIRECTION ( 'NONE',  ( -0.000000000000000000, -0.000000000000000000, 1.000000000000000000 ) ) ;
#6920=FACE_OUTER_BOUND ( 'NONE', #2377, .T. ) ;
#6921=DIRECTION ( 'NONE',  ( 1.000000000000000000, 0.000000000000000000, 0.000000000000000000 ) ) ;
#6928=ORIENTED_EDGE ( 'NONE', *, *, #5812, .F. ) ;
#6931=ORIENTED_EDGE ( 'NONE', *, *, #354, .T. ) ;
#6940=ORIENTED_EDGE ( 'NONE', *, *, #3073, .F. ) ;
#6945=CARTESIAN_POINT ( 'NONE',  ( -63.51644452187067458, 49.96174644486002592, 10.00000000000000000 ) ) ;
#6959=EDGE_CURVE ( 'NONE', #1194, #5183, #6711, .T. ) ;
#6966=CIRCLE ( 'NONE', #4063, 5.250000000000000888 ) ;
#6970=EDGE_CURVE ( 'NONE', #1194, #1572, #5284, .T. ) ;
#6976=ADVANCED_FACE ( 'NONE', ( #6321 ), #7569, .F. ) ;
#6985=CARTESIAN_POINT ( 'NONE',  ( 21.01644452187122170, -80.83980388508783221, 0.000000000000000000 ) ) ;
#6999=CYLINDRICAL_SURFACE ( 'NONE', #1884, 5.250000000000004441 ) ;
#7012=ORIENTED_EDGE ( 'NONE', *, *, #2415, .T. ) ;
#7023=ORIENTED_EDGE ( 'NONE', *, *, #1339, .F. ) ;
#7027=DIRECTION ( 'NONE',  ( 1.000000000000000000, 0.000000000000000000, 0.000000000000000000 ) ) ;
#7028=CARTESIAN_POINT ( 'NONE',  ( 31.51644452187122525, -80.83980388508783221, 0.000000000000000000 ) ) ;
#7030=VECTOR ( 'NONE', #4186, 1000.000000000000000 ) ;
#7032=ORIENTED_EDGE ( 'NONE', *, *, #3309, .T. ) ;
#7033=VERTEX_POINT ( 'NONE', #146 ) ;
#7034=AXIS2_PLACEMENT_3D ( 'NONE', #1244, #6098, #4872 ) ;
#7035=CARTESIAN_POINT ( 'NONE',  ( -63.51644452187023404, -49.96174644486060856, 10.00000000000000000 ) ) ;
#7040=EDGE_CURVE ( 'NONE', #6086, #294, #2577, .T. ) ;
#7047=DIRECTION ( 'NONE',  ( 1.000000000000000000, 0.000000000000000000, 0.000000000000000000 ) ) ;
#7060=DIRECTION ( 'NONE',  ( 0.000000000000000000, 0.000000000000000000, 1.000000000000000000 ) ) ;
#7075=DIRECTION ( 'NONE',  ( 0.5000000000000101030, -0.8660254037844328234, 0.000000000000000000 ) ) ;
#7076=EDGE_CURVE ( 'NONE', #4919, #6651, #6966, .T. ) ;
#7086=CYLINDRICAL_SURFACE ( 'NONE', #4749, 40.00000000000000711 ) ;
#7089=CYLINDRICAL_SURFACE ( 'NONE', #2019, 150.0000000000000568 ) ;
#7096=AXIS2_PLACEMENT_3D ( 'NONE', #7100, #104, #4324 ) ;
#7097=CYLINDRICAL_SURFACE ( 'NONE', #6315, 150.0000000000000568 ) ;
#7098=DIRECTION ( 'NONE',  ( -0.000000000000000000, -0.000000000000000000, 1.000000000000000000 ) ) ;
#7099=DIRECTION ( 'NONE',  ( -1.000000000000000000, 0.000000000000000000, 0.000000000000000000 ) ) ;
#7100=CARTESIAN_POINT ( 'NONE',  ( -68.76644452187068168, 49.96174644486002592, 10.00000000000000000 ) ) ;
#7119=DIRECTION ( 'NONE',  ( -0.000000000000000000, -0.000000000000000000, 1.000000000000000000 ) ) ;
#7121=EDGE_CURVE ( 'NONE', #7440, #5822, #407, .T. ) ;
#7133=CARTESIAN_POINT ( 'NONE',  ( 0.000000000000000000, 0.000000000000000000, 10.00000000000000000 ) ) ;
#7137=ORIENTED_EDGE ( 'NONE', *, *, #7450, .T. ) ;
#7143=CIRCLE ( 'NONE', #964, 5.250000000000004441 ) ;
#7144=CARTESIAN_POINT ( 'NONE',  ( 26.26644452187053957, 80.83980388508807380, 10.00000000000000000 ) ) ;
#7150=VERTEX_POINT ( 'NONE', #3382 ) ;
#7174=CIRCLE ( 'NONE', #5024, 150.0000000000000568 ) ;
#7189=CARTESIAN_POINT ( 'NONE',  ( -145.1064334105735725, 38.00161816110973234, 5.000000000000000000 ) ) ;
#7192=ORIENTED_EDGE ( 'NONE', *, *, #2590, .T. ) ;
#7204=EDGE_CURVE ( 'NONE', #6340, #3290, #7721, .T. ) ;
#7209=LINE ( 'NONE', #3624, #2770 ) ;
#7212=ORIENTED_EDGE ( 'NONE', *, *, #894, .T. ) ;
#7223=EDGE_CURVE ( 'NONE', #5511, #6752, #6463, .T. ) ;
#7224=EDGE_LOOP ( 'NONE', ( #4596, #4611, #1940, #663 ) ) ;
#7235=VECTOR ( 'NONE', #4579, 1000.000000000000000 ) ;
#7249=( NAMED_UNIT ( * ) SI_UNIT ( $, .STERADIAN. ) SOLID_ANGLE_UNIT ( ) );
#7260=VERTEX_POINT ( 'NONE', #4823 ) ;
#7274=FACE_OUTER_BOUND ( 'NONE', #4372, .T. ) ;
#7280=ORIENTED_EDGE ( 'NONE', *, *, #3497, .F. ) ;
#7284=CARTESIAN_POINT ( 'NONE',  ( -105.4635834177236546, -106.6650485055571380, 0.000000000000000000 ) ) ;
#7312=FACE_OUTER_BOUND ( 'NONE', #106, .T. ) ;
#7313=CIRCLE ( 'NONE', #4661, 150.0000000000000568 ) ;
#7315=DIRECTION ( 'NONE',  ( 0.000000000000000000, 0.000000000000000000, 1.000000000000000000 ) ) ;
#7321=ADVANCED_FACE ( 'NONE', ( #7312 ), #5570, .T. ) ;
#7322=AXIS2_PLACEMENT_3D ( 'NONE', #495, #1163, #7047 ) ;
#7323=CYLINDRICAL_SURFACE ( 'NONE', #5559, 40.00000000000000711 ) ;
#7335=DIRECTION ( 'NONE',  ( 0.000000000000000000, -0.000000000000000000, -1.000000000000000000 ) ) ;
#7338=VERTEX_POINT ( 'NONE', #721 ) ;
#7353=CARTESIAN_POINT ( 'NONE',  ( -68.76644452187024115, -49.96174644486060856, 10.00000000000000000 ) ) ;
#7358=DIRECTION ( 'NONE',  ( 1.000000000000000000, 0.000000000000000000, 0.000000000000000000 ) ) ;
#7360=CARTESIAN_POINT ( 'NONE',  ( 129.9038105676649764, 75.00000000000153477, 10.00000000000000000 ) ) ;
#7366=CARTESIAN_POINT ( 'NONE',  ( 0.000000000000000000, 0.000000000000000000, 10.00000000000000000 ) ) ;
#7369=EDGE_CURVE ( 'NONE', #1526, #989, #6605, .T. ) ;
#7379=CARTESIAN_POINT ( 'NONE',  ( 0.000000000000000000, 0.000000000000000000, 0.000000000000000000 ) ) ;
#7391=FACE_BOUND ( 'NONE', #2038, .T. ) ;
#7417=ADVANCED_FACE ( 'NONE', ( #7274 ), #4386, .F. ) ;
#7418=LINE ( 'NONE', #3831, #3387 ) ;
#7427=DIRECTION ( 'NONE',  ( 0.000000000000000000, 0.000000000000000000, -1.000000000000000000 ) ) ;
#7430=AXIS2_PLACEMENT_3D ( 'NONE', #3201, #2764, #5009 ) ;
#7432=DIRECTION ( 'NONE',  ( -0.000000000000000000, -0.000000000000000000, 1.000000000000000000 ) ) ;
#7440=VERTEX_POINT ( 'NONE', #3912 ) ;
#7442=AXIS2_PLACEMENT_3D ( 'NONE', #6665, #6076, #664 ) ;
#7443=FACE_OUTER_BOUND ( 'NONE', #6347, .T. ) ;
#7444=LINE ( 'NONE', #1006, #6676 ) ;
#7448=EDGE_CURVE ( 'NONE', #7150, #989, #4968, .T. ) ;
#7450=EDGE_CURVE ( 'NONE', #7260, #5121, #5843, .T. ) ;
#7459=EDGE_CURVE ( 'NONE', #57, #4452, #3988, .T. ) ;
#7467=FACE_BOUND ( 'NONE', #1254, .T. ) ;
#7468=AXIS2_PLACEMENT_3D ( 'NONE', #3983, #7529, #5798 ) ;
#7469=CYLINDRICAL_SURFACE ( 'NONE', #949, 30.00000000000000000 ) ;
#7477=ORIENTED_EDGE ( 'NONE', *, *, #6643, .F. ) ;
#7478=VERTEX_POINT ( 'NONE', #2150 ) ;
#7483=DIRECTION ( 'NONE',  ( -1.000000000000000000, 0.000000000000000000, 0.000000000000000000 ) ) ;
#7485=AXIS2_PLACEMENT_3D ( 'NONE', #1301, #3758, #5977 ) ;
#7486=ORIENTED_EDGE ( 'NONE', *, *, #938, .F. ) ;
#7488=DIRECTION ( 'NONE',  ( 1.000000000000000000, 0.000000000000000000, 0.000000000000000000 ) ) ;
#7494=DIRECTION ( 'NONE',  ( 0.000000000000000000, 0.000000000000000000, 1.000000000000000000 ) ) ;
#7501=VECTOR ( 'NONE', #1421, 1000.000000000000000 ) ;
#7505=CYLINDRICAL_SURFACE ( 'NONE', #6797, 5.250000000000000888 ) ;
#7508=AXIS2_PLACEMENT_3D ( 'NONE', #3555, #1752, #2970 ) ;
#7512=ORIENTED_EDGE ( 'NONE', *, *, #1278, .T. ) ;
#7517=DIRECTION ( 'NONE',  ( 1.000000000000000000, 0.000000000000000000, 0.000000000000000000 ) ) ;
#7524=CIRCLE ( 'NONE', #2131, 5.250000000000000888 ) ;
#7528=DIRECTION ( 'NONE',  ( 0.000000000000000000, 0.000000000000000000, 1.000000000000000000 ) ) ;
#7529=DIRECTION ( 'NONE',  ( 0.000000000000000000, 0.000000000000000000, -1.000000000000000000 ) ) ;
#7532=ADVANCED_FACE ( 'NONE', ( #5168 ), #3287, .T. ) ;
#7534=DIRECTION ( 'NONE',  ( -1.000000000000000000, 0.000000000000000000, 0.000000000000000000 ) ) ;
#7546=DIRECTION ( 'NONE',  ( -0.000000000000000000, -0.000000000000000000, 1.000000000000000000 ) ) ;
#7549=EDGE_CURVE ( 'NONE', #4996, #6340, #1585, .T. ) ;
#7552=ORIENTED_EDGE ( 'NONE', *, *, #2848, .F. ) ;
#7560=DIRECTION ( 'NONE',  ( 0.000000000000000000, 0.000000000000000000, 1.000000000000000000 ) ) ;
#7569=CYLINDRICAL_SURFACE ( 'NONE', #7468, 40.00000000000000711 ) ;
#7571=CARTESIAN_POINT ( 'NONE',  ( -145.1064334105733451, -38.00161816111073421, 10.00000000000000000 ) ) ;
#7600=EDGE_LOOP ( 'NONE', ( #195, #7192, #6894, #4057 ) ) ;
#7606=CARTESIAN_POINT ( 'NONE',  ( -150.0000000000000568, 0.000000000000000000, 0.000000000000000000 ) ) ;
#7614=CARTESIAN_POINT ( 'NONE',  ( -150.0000000000000568, 0.000000000000000000, 10.00000000000000000 ) ) ;
#7616=CARTESIAN_POINT ( 'NONE',  ( 0.000000000000000000, 0.000000000000000000, 0.000000000000000000 ) ) ;
#7622=DIRECTION ( 'NONE',  ( 0.000000000000000000, 0.000000000000000000, 1.000000000000000000 ) ) ;
#7627=ORIENTED_EDGE ( 'NONE', *, *, #5103, .F. ) ;
#7628=VECTOR ( 'NONE', #1761, 1000.000000000000000 ) ;
#7632=DIRECTION ( 'NONE',  ( -0.000000000000000000, -0.000000000000000000, 1.000000000000000000 ) ) ;
#7635=LINE ( 'NONE', #497, #5881 ) ;
#7639=ORIENTED_EDGE ( 'NONE', *, *, #2081, .T. ) ;
#7648=CARTESIAN_POINT ( 'NONE',  ( 21.01644452187054313, 80.83980388508807380, 10.00000000000000000 ) ) ;
#7650=CIRCLE ( 'NONE', #6399, 40.00000000000000000 ) ;
#7651=ADVANCED_FACE ( 'NONE', ( #3885 ), #1476, .T. ) ;
#7659=ORIENTED_EDGE ( 'NONE', *, *, #215, .F. ) ;
#7660=CIRCLE ( 'NONE', #7034, 5.250000000000004441 ) ;
#7682=AXIS2_PLACEMENT_3D ( 'NONE', #6830, #4534, #827 ) ;
#7694=CARTESIAN_POINT ( 'NONE',  ( -39.64284999284935651, -144.6666666666667140, 0.000000000000000000 ) ) ;
#7702=CIRCLE ( 'NONE', #23, 5.250000000000004441 ) ;
#7716=CARTESIAN_POINT ( 'NONE',  ( 90.25000000000001421, 9.720002580593245511E-13, 10.00000000000000000 ) ) ;
#7721=CIRCLE ( 'NONE', #2066, 40.00000000000001421 ) ;
#7733=DIRECTION ( 'NONE',  ( -0.000000000000000000, -0.000000000000000000, 1.000000000000000000 ) ) ;
#7734=ORIENTED_EDGE ( 'NONE', *, *, #7448, .T. ) ;
#7736=EDGE_LOOP ( 'NONE', ( #7552, #5498, #4690, #5412 ) ) ;
#7738=ORIENTED_EDGE ( 'NONE', *, *, #215, .T. ) ;
#7741=FACE_OUTER_BOUND ( 'NONE', #3240, .T. ) ;
#7817=COLOUR_RGB('Sky Blue',0.24,0.69,0.87);
#7818=FILL_AREA_STYLE_COLOUR('',#7817);
#7819=FILL_AREA_STYLE('',(#7818));
#7820=SURFACE_STYLE_FILL_AREA(#7819);
#7821=SURFACE_SIDE_STYLE('',(#7820));
#7822=SURFACE_STYLE_USAGE(.BOTH.,#7821);
#7823=PRESENTATION_STYLE_ASSIGNMENT((#7822));
ENDSEC;
END-ISO-10303-21;
